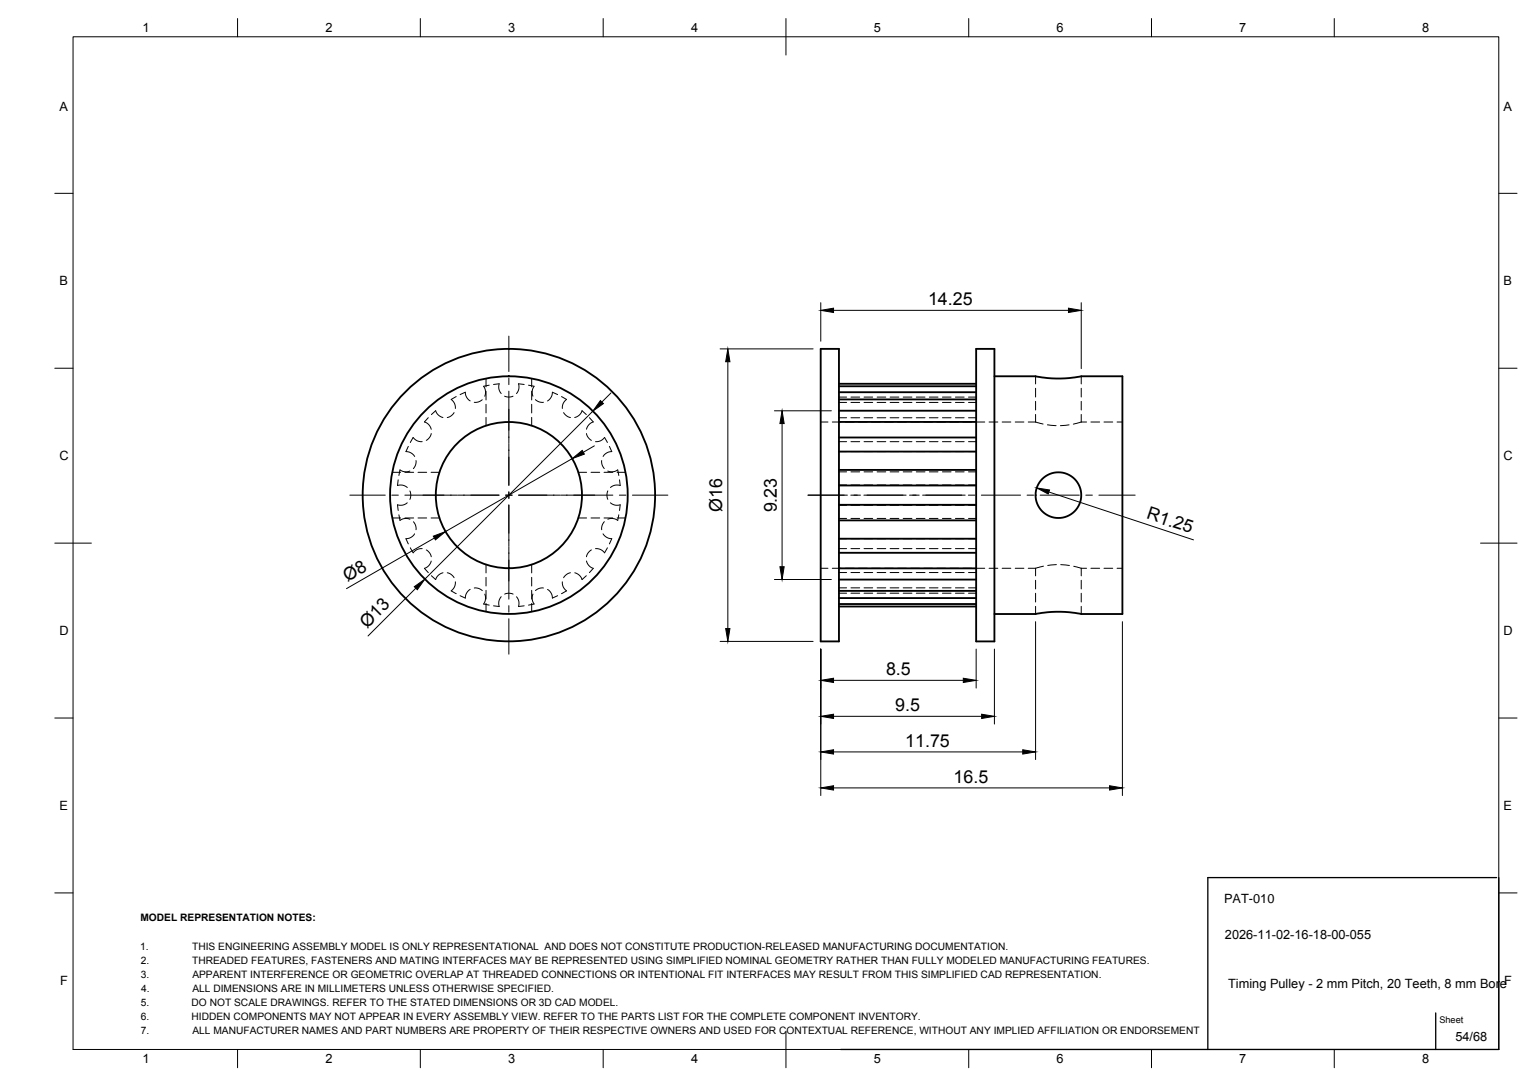
ISO-10303-21;
HEADER;
/* Generated by software containing ST-Developer
 * from STEP Tools, Inc. (www.steptools.com) 
 */

FILE_DESCRIPTION(
/* description */ ('Belt conveyor head drive unit'),
/* implementation_level */ '2;1');

FILE_NAME(
/* name */ 'Timing Pulley - 2 mm Pitch, 20 Teeth, 8 mm Bore.step',
/* time_stamp */ '2026-10-28T03:26:19-07:00',
/* author */ (''),
/* organization */ (''),
/* preprocessor_version */ 'ST-DEVELOPER v20.2',
/* originating_system */ 'Autodesk Translation Framework v15.17.0.0',
/* authorisation */ '');

FILE_SCHEMA (('AUTOMOTIVE_DESIGN { 1 0 10303 214 3 1 1 }'));
ENDSEC;

DATA;
#10=MECHANICAL_DESIGN_GEOMETRIC_PRESENTATION_REPRESENTATION('',(#915),#27069);
#585=B_SPLINE_CURVE_WITH_KNOTS('',3,(#24720,#24721,#24722,#24723,#24724,
#24725,#24726,#24727,#24728,#24729),.UNSPECIFIED.,.F.,.F.,(4,2,2,2,4),(0.566550474129931,
0.613761886174531,0.66097329821913,0.708186965196186,0.755400632173242),
 .UNSPECIFIED.);
#586=B_SPLINE_CURVE_WITH_KNOTS('',3,(#24731,#24732,#24733,#24734,#24735,
#24736,#24737,#24738,#24739,#24740,#24741,#24742,#24743,#24744,#24745,#24746,
#24747,#24748),.UNSPECIFIED.,.F.,.F.,(4,2,2,2,2,2,2,2,4),(0.18885015804331,
0.23606157008791,0.283272982132509,0.330486649109565,0.377700316086621,
0.424913983063677,0.472127650040732,0.519339062085332,0.566550474129931),
 .UNSPECIFIED.);
#587=B_SPLINE_CURVE_WITH_KNOTS('',3,(#24749,#24750,#24751,#24752,#24753,
#24754,#24755,#24756,#24757,#24758),.UNSPECIFIED.,.F.,.F.,(4,2,2,2,4),(0.755400632173242,
0.802614299150298,0.849827966127353,0.897039378171953,0.944250790216552),
 .UNSPECIFIED.);
#588=B_SPLINE_CURVE_WITH_KNOTS('',3,(#24762,#24763,#24764,#24765,#24766,
#24767,#24768,#24769,#24770,#24771),.UNSPECIFIED.,.F.,.F.,(4,2,2,2,4),(0.189723673274825,
0.237146208024627,0.28456874277443,0.33200804466204,0.37944734654965),
 .UNSPECIFIED.);
#589=B_SPLINE_CURVE_WITH_KNOTS('',3,(#24773,#24774,#24775,#24776,#24777,
#24778,#24779,#24780,#24781,#24782),.UNSPECIFIED.,.F.,.F.,(4,2,2,2,4),(0.,
0.0474393018876097,0.0948786037752193,0.142301138525022,0.189723673274825),
 .UNSPECIFIED.);
#590=B_SPLINE_CURVE_WITH_KNOTS('',3,(#24784,#24785,#24786,#24787,#24788,
#24789,#24790,#24791,#24792,#24793),.UNSPECIFIED.,.F.,.F.,(4,2,2,2,4),(0.569171019824474,
0.616593554574277,0.66401608932408,0.711455391211689,0.758894693099299),
 .UNSPECIFIED.);
#591=B_SPLINE_CURVE_WITH_KNOTS('',3,(#24794,#24795,#24796,#24797,#24798,
#24799,#24800,#24801,#24802,#24803),.UNSPECIFIED.,.F.,.F.,(4,2,2,2,4),(0.37944734654965,
0.426886648437259,0.474325950324869,0.521748485074671,0.569171019824474),
 .UNSPECIFIED.);
#592=B_SPLINE_CURVE_WITH_KNOTS('',3,(#24807,#24808,#24809,#24810,#24811,
#24812,#24813,#24814,#24815,#24816,#24817,#24818,#24819,#24820,#24821,#24822,
#24823,#24824),.UNSPECIFIED.,.F.,.F.,(4,2,2,2,2,2,2,2,4),(0.,0.0474393018876097,
0.0948786037752194,0.142301138525022,0.189723673274825,0.237146208024628,
0.28456874277443,0.33200804466204,0.37944734654965),.UNSPECIFIED.);
#593=B_SPLINE_CURVE_WITH_KNOTS('',3,(#24825,#24826,#24827,#24828,#24829,
#24830,#24831,#24832,#24833,#24834,#24835,#24836,#24837,#24838,#24839,#24840,
#24841,#24842),.UNSPECIFIED.,.F.,.F.,(4,2,2,2,2,2,2,2,4),(0.37944734654965,
0.426886648437259,0.474325950324869,0.521748485074672,0.569171019824474,
0.616593554574277,0.66401608932408,0.711455391211689,0.758894693099299),
 .UNSPECIFIED.);
#594=B_SPLINE_CURVE_WITH_KNOTS('',3,(#24846,#24847,#24848,#24849,#24850,
#24851,#24852,#24853,#24854,#24855),.UNSPECIFIED.,.F.,.F.,(4,2,2,2,4),(0.566550474129931,
0.613761886174531,0.66097329821913,0.708186965196186,0.755400632173242),
 .UNSPECIFIED.);
#595=B_SPLINE_CURVE_WITH_KNOTS('',3,(#24857,#24858,#24859,#24860,#24861,
#24862,#24863,#24864,#24865,#24866,#24867,#24868,#24869,#24870,#24871,#24872,
#24873,#24874),.UNSPECIFIED.,.F.,.F.,(4,2,2,2,2,2,2,2,4),(0.188850158043311,
0.23606157008791,0.283272982132509,0.330486649109565,0.377700316086621,
0.424913983063677,0.472127650040733,0.519339062085332,0.566550474129931),
 .UNSPECIFIED.);
#596=B_SPLINE_CURVE_WITH_KNOTS('',3,(#24875,#24876,#24877,#24878,#24879,
#24880,#24881,#24882,#24883,#24884),.UNSPECIFIED.,.F.,.F.,(4,2,2,2,4),(0.755400632173242,
0.802614299150298,0.849827966127354,0.897039378171953,0.944250790216552),
 .UNSPECIFIED.);
#597=B_SPLINE_CURVE_WITH_KNOTS('',3,(#24894,#24895,#24896,#24897,#24898,
#24899,#24900,#24901,#24902,#24903,#24904,#24905,#24906,#24907,#24908,#24909,
#24910,#24911),.UNSPECIFIED.,.F.,.F.,(4,2,2,2,2,2,2,2,4),(0.18885015804331,
0.23606157008791,0.283272982132509,0.330486649109565,0.377700316086621,
0.424913983063677,0.472127650040732,0.519339062085332,0.566550474129931),
 .UNSPECIFIED.);
#598=B_SPLINE_CURVE_WITH_KNOTS('',3,(#24913,#24914,#24915,#24916,#24917,
#24918,#24919,#24920,#24921,#24922),.UNSPECIFIED.,.F.,.F.,(4,2,2,2,4),(0.566550474129931,
0.613761886174531,0.66097329821913,0.708186965196186,0.755400632173242),
 .UNSPECIFIED.);
#599=B_SPLINE_CURVE_WITH_KNOTS('',3,(#24923,#24924,#24925,#24926,#24927,
#24928,#24929,#24930,#24931,#24932),.UNSPECIFIED.,.F.,.F.,(4,2,2,2,4),(0.755400632173242,
0.802614299150298,0.849827966127353,0.897039378171953,0.944250790216552),
 .UNSPECIFIED.);
#600=B_SPLINE_CURVE_WITH_KNOTS('',3,(#24935,#24936,#24937,#24938,#24939,
#24940,#24941,#24942,#24943,#24944,#24945,#24946,#24947,#24948,#24949,#24950,
#24951,#24952),.UNSPECIFIED.,.F.,.F.,(4,2,2,2,2,2,2,2,4),(0.188850158043311,
0.23606157008791,0.283272982132509,0.330486649109565,0.377700316086621,
0.424913983063677,0.472127650040733,0.519339062085332,0.566550474129932),
 .UNSPECIFIED.);
#601=B_SPLINE_CURVE_WITH_KNOTS('',3,(#24954,#24955,#24956,#24957,#24958,
#24959,#24960,#24961,#24962,#24963),.UNSPECIFIED.,.F.,.F.,(4,2,2,2,4),(0.566550474129932,
0.613761886174531,0.66097329821913,0.708186965196186,0.755400632173242),
 .UNSPECIFIED.);
#602=B_SPLINE_CURVE_WITH_KNOTS('',3,(#24964,#24965,#24966,#24967,#24968,
#24969,#24970,#24971,#24972,#24973),.UNSPECIFIED.,.F.,.F.,(4,2,2,2,4),(0.755400632173242,
0.802614299150298,0.849827966127354,0.897039378171953,0.944250790216552),
 .UNSPECIFIED.);
#603=B_SPLINE_CURVE_WITH_KNOTS('',3,(#24978,#24979,#24980,#24981,#24982,
#24983,#24984,#24985,#24986,#24987,#24988,#24989,#24990,#24991,#24992,#24993,
#24994,#24995),.UNSPECIFIED.,.F.,.F.,(4,2,2,2,2,2,2,2,4),(0.,0.0474393018876097,
0.0948786037752193,0.142301138525022,0.189723673274825,0.237146208024627,
0.28456874277443,0.33200804466204,0.37944734654965),.UNSPECIFIED.);
#604=B_SPLINE_CURVE_WITH_KNOTS('',3,(#24996,#24997,#24998,#24999,#25000,
#25001,#25002,#25003,#25004,#25005,#25006,#25007,#25008,#25009,#25010,#25011,
#25012,#25013),.UNSPECIFIED.,.F.,.F.,(4,2,2,2,2,2,2,2,4),(0.37944734654965,
0.426886648437259,0.474325950324869,0.521748485074672,0.569171019824474,
0.616593554574277,0.66401608932408,0.711455391211689,0.758894693099299),
 .UNSPECIFIED.);
#605=B_SPLINE_CURVE_WITH_KNOTS('',3,(#25017,#25018,#25019,#25020,#25021,
#25022,#25023,#25024,#25025,#25026,#25027,#25028,#25029,#25030,#25031,#25032,
#25033,#25034),.UNSPECIFIED.,.F.,.F.,(4,2,2,2,2,2,2,2,4),(0.,0.0474393018876097,
0.0948786037752194,0.142301138525022,0.189723673274825,0.237146208024627,
0.28456874277443,0.33200804466204,0.37944734654965),.UNSPECIFIED.);
#606=B_SPLINE_CURVE_WITH_KNOTS('',3,(#25035,#25036,#25037,#25038,#25039,
#25040,#25041,#25042,#25043,#25044,#25045,#25046,#25047,#25048,#25049,#25050,
#25051,#25052),.UNSPECIFIED.,.F.,.F.,(4,2,2,2,2,2,2,2,4),(0.37944734654965,
0.426886648437259,0.474325950324869,0.521748485074672,0.569171019824474,
0.616593554574277,0.66401608932408,0.711455391211689,0.758894693099299),
 .UNSPECIFIED.);
#761=SHAPE_REPRESENTATION_RELATIONSHIP('SRR','None',#27409,#830);
#830=ADVANCED_BREP_SHAPE_REPRESENTATION('',(#996),#27051);
#915=STYLED_ITEM('',(#27811),#996);
#996=MANIFOLD_SOLID_BREP('Body1',#13784);
#1222=FACE_BOUND('',#3204,.T.);
#1223=FACE_BOUND('',#3205,.T.);
#1224=FACE_BOUND('',#3206,.T.);
#1225=FACE_BOUND('',#3210,.T.);
#1226=FACE_BOUND('',#3211,.T.);
#1227=FACE_BOUND('',#3212,.T.);
#1228=FACE_BOUND('',#3214,.T.);
#1229=FACE_BOUND('',#3216,.T.);
#1230=FACE_BOUND('',#3219,.T.);
#1231=FACE_BOUND('',#3221,.T.);
#1232=FACE_BOUND('',#3224,.T.);
#1566=PLANE('',#15740);
#1567=PLANE('',#15741);
#1568=PLANE('',#15785);
#1569=PLANE('',#15786);
#1570=PLANE('',#15830);
#2191=FACE_OUTER_BOUND('',#3201,.T.);
#2192=FACE_OUTER_BOUND('',#3202,.T.);
#2193=FACE_OUTER_BOUND('',#3203,.T.);
#2194=FACE_OUTER_BOUND('',#3207,.T.);
#2195=FACE_OUTER_BOUND('',#3208,.T.);
#2196=FACE_OUTER_BOUND('',#3209,.T.);
#2197=FACE_OUTER_BOUND('',#3213,.T.);
#2198=FACE_OUTER_BOUND('',#3215,.T.);
#2199=FACE_OUTER_BOUND('',#3217,.T.);
#2200=FACE_OUTER_BOUND('',#3218,.T.);
#2201=FACE_OUTER_BOUND('',#3220,.T.);
#2202=FACE_OUTER_BOUND('',#3222,.T.);
#2203=FACE_OUTER_BOUND('',#3223,.T.);
#2204=FACE_OUTER_BOUND('',#3225,.T.);
#2205=FACE_OUTER_BOUND('',#3226,.T.);
#2206=FACE_OUTER_BOUND('',#3227,.T.);
#2207=FACE_OUTER_BOUND('',#3228,.T.);
#2208=FACE_OUTER_BOUND('',#3229,.T.);
#2209=FACE_OUTER_BOUND('',#3230,.T.);
#2210=FACE_OUTER_BOUND('',#3231,.T.);
#2211=FACE_OUTER_BOUND('',#3232,.T.);
#2212=FACE_OUTER_BOUND('',#3233,.T.);
#2213=FACE_OUTER_BOUND('',#3234,.T.);
#2214=FACE_OUTER_BOUND('',#3235,.T.);
#2215=FACE_OUTER_BOUND('',#3236,.T.);
#2216=FACE_OUTER_BOUND('',#3237,.T.);
#2217=FACE_OUTER_BOUND('',#3238,.T.);
#2218=FACE_OUTER_BOUND('',#3239,.T.);
#2219=FACE_OUTER_BOUND('',#3240,.T.);
#2220=FACE_OUTER_BOUND('',#3241,.T.);
#2221=FACE_OUTER_BOUND('',#3242,.T.);
#2222=FACE_OUTER_BOUND('',#3243,.T.);
#2223=FACE_OUTER_BOUND('',#3244,.T.);
#2224=FACE_OUTER_BOUND('',#3245,.T.);
#2225=FACE_OUTER_BOUND('',#3246,.T.);
#2226=FACE_OUTER_BOUND('',#3247,.T.);
#2227=FACE_OUTER_BOUND('',#3248,.T.);
#2228=FACE_OUTER_BOUND('',#3249,.T.);
#2229=FACE_OUTER_BOUND('',#3250,.T.);
#2230=FACE_OUTER_BOUND('',#3251,.T.);
#2231=FACE_OUTER_BOUND('',#3252,.T.);
#2232=FACE_OUTER_BOUND('',#3253,.T.);
#2233=FACE_OUTER_BOUND('',#3254,.T.);
#2234=FACE_OUTER_BOUND('',#3255,.T.);
#2235=FACE_OUTER_BOUND('',#3256,.T.);
#2236=FACE_OUTER_BOUND('',#3257,.T.);
#2237=FACE_OUTER_BOUND('',#3258,.T.);
#2238=FACE_OUTER_BOUND('',#3259,.T.);
#2239=FACE_OUTER_BOUND('',#3260,.T.);
#2240=FACE_OUTER_BOUND('',#3261,.T.);
#2241=FACE_OUTER_BOUND('',#3262,.T.);
#2242=FACE_OUTER_BOUND('',#3263,.T.);
#2243=FACE_OUTER_BOUND('',#3264,.T.);
#3201=EDGE_LOOP('',(#11302,#11303,#11304,#11305,#11306,#11307,#11308,#11309,
#11310));
#3202=EDGE_LOOP('',(#11311,#11312,#11313,#11314,#11315,#11316,#11317));
#3203=EDGE_LOOP('',(#11318,#11319,#11320,#11321,#11322,#11323,#11324,#11325,
#11326));
#3204=EDGE_LOOP('',(#11327,#11328,#11329));
#3205=EDGE_LOOP('',(#11330,#11331,#11332));
#3206=EDGE_LOOP('',(#11333,#11334,#11335));
#3207=EDGE_LOOP('',(#11336,#11337,#11338,#11339,#11340,#11341,#11342));
#3208=EDGE_LOOP('',(#11343,#11344,#11345,#11346,#11347,#11348,#11349));
#3209=EDGE_LOOP('',(#11350,#11351,#11352,#11353,#11354,#11355,#11356,#11357,
#11358,#11359));
#3210=EDGE_LOOP('',(#11360,#11361));
#3211=EDGE_LOOP('',(#11362,#11363));
#3212=EDGE_LOOP('',(#11364,#11365));
#3213=EDGE_LOOP('',(#11366));
#3214=EDGE_LOOP('',(#11367));
#3215=EDGE_LOOP('',(#11368));
#3216=EDGE_LOOP('',(#11369,#11370,#11371,#11372,#11373,#11374,#11375,#11376,
#11377,#11378,#11379,#11380,#11381,#11382,#11383,#11384,#11385,#11386,#11387,
#11388,#11389,#11390,#11391,#11392,#11393,#11394,#11395,#11396,#11397,#11398,
#11399,#11400,#11401,#11402,#11403,#11404,#11405,#11406,#11407,#11408));
#3217=EDGE_LOOP('',(#11409,#11410,#11411,#11412));
#3218=EDGE_LOOP('',(#11413));
#3219=EDGE_LOOP('',(#11414));
#3220=EDGE_LOOP('',(#11415));
#3221=EDGE_LOOP('',(#11416,#11417,#11418,#11419,#11420,#11421,#11422,#11423,
#11424,#11425,#11426,#11427,#11428,#11429,#11430,#11431,#11432,#11433,#11434,
#11435,#11436,#11437,#11438,#11439,#11440,#11441,#11442,#11443,#11444,#11445,
#11446,#11447,#11448,#11449,#11450,#11451,#11452,#11453,#11454,#11455));
#3222=EDGE_LOOP('',(#11456,#11457,#11458,#11459));
#3223=EDGE_LOOP('',(#11460));
#3224=EDGE_LOOP('',(#11461));
#3225=EDGE_LOOP('',(#11462,#11463,#11464,#11465));
#3226=EDGE_LOOP('',(#11466,#11467,#11468,#11469));
#3227=EDGE_LOOP('',(#11470,#11471,#11472,#11473));
#3228=EDGE_LOOP('',(#11474,#11475,#11476,#11477));
#3229=EDGE_LOOP('',(#11478,#11479,#11480,#11481));
#3230=EDGE_LOOP('',(#11482,#11483,#11484,#11485));
#3231=EDGE_LOOP('',(#11486,#11487,#11488,#11489));
#3232=EDGE_LOOP('',(#11490,#11491,#11492,#11493));
#3233=EDGE_LOOP('',(#11494,#11495,#11496,#11497));
#3234=EDGE_LOOP('',(#11498,#11499,#11500,#11501));
#3235=EDGE_LOOP('',(#11502,#11503,#11504,#11505));
#3236=EDGE_LOOP('',(#11506,#11507,#11508,#11509));
#3237=EDGE_LOOP('',(#11510,#11511,#11512,#11513));
#3238=EDGE_LOOP('',(#11514,#11515,#11516,#11517));
#3239=EDGE_LOOP('',(#11518,#11519,#11520,#11521));
#3240=EDGE_LOOP('',(#11522,#11523,#11524,#11525));
#3241=EDGE_LOOP('',(#11526,#11527,#11528,#11529));
#3242=EDGE_LOOP('',(#11530,#11531,#11532,#11533));
#3243=EDGE_LOOP('',(#11534,#11535,#11536,#11537));
#3244=EDGE_LOOP('',(#11538,#11539,#11540,#11541));
#3245=EDGE_LOOP('',(#11542,#11543,#11544,#11545));
#3246=EDGE_LOOP('',(#11546,#11547,#11548,#11549));
#3247=EDGE_LOOP('',(#11550,#11551,#11552,#11553));
#3248=EDGE_LOOP('',(#11554,#11555,#11556,#11557));
#3249=EDGE_LOOP('',(#11558,#11559,#11560,#11561));
#3250=EDGE_LOOP('',(#11562,#11563,#11564,#11565));
#3251=EDGE_LOOP('',(#11566,#11567,#11568,#11569));
#3252=EDGE_LOOP('',(#11570,#11571,#11572,#11573));
#3253=EDGE_LOOP('',(#11574,#11575,#11576,#11577));
#3254=EDGE_LOOP('',(#11578,#11579,#11580,#11581));
#3255=EDGE_LOOP('',(#11582,#11583,#11584,#11585));
#3256=EDGE_LOOP('',(#11586,#11587,#11588,#11589));
#3257=EDGE_LOOP('',(#11590,#11591,#11592,#11593));
#3258=EDGE_LOOP('',(#11594,#11595,#11596,#11597));
#3259=EDGE_LOOP('',(#11598,#11599,#11600,#11601));
#3260=EDGE_LOOP('',(#11602,#11603,#11604,#11605));
#3261=EDGE_LOOP('',(#11606,#11607,#11608,#11609));
#3262=EDGE_LOOP('',(#11610,#11611,#11612,#11613));
#3263=EDGE_LOOP('',(#11614,#11615,#11616,#11617));
#3264=EDGE_LOOP('',(#11618,#11619,#11620,#11621));
#4067=LINE('',#24760,#4859);
#4068=LINE('',#24844,#4860);
#4069=LINE('',#24888,#4861);
#4070=LINE('',#24890,#4862);
#4071=LINE('',#24976,#4863);
#4072=LINE('',#25053,#4864);
#4073=LINE('',#25057,#4865);
#4074=LINE('',#25059,#4866);
#4075=LINE('',#25148,#4867);
#4076=LINE('',#25236,#4868);
#4077=LINE('',#25239,#4869);
#4078=LINE('',#25240,#4870);
#4079=LINE('',#25242,#4871);
#4080=LINE('',#25244,#4872);
#4081=LINE('',#25246,#4873);
#4082=LINE('',#25248,#4874);
#4083=LINE('',#25250,#4875);
#4084=LINE('',#25252,#4876);
#4085=LINE('',#25254,#4877);
#4086=LINE('',#25256,#4878);
#4087=LINE('',#25258,#4879);
#4088=LINE('',#25260,#4880);
#4089=LINE('',#25262,#4881);
#4090=LINE('',#25264,#4882);
#4091=LINE('',#25266,#4883);
#4092=LINE('',#25268,#4884);
#4093=LINE('',#25270,#4885);
#4094=LINE('',#25272,#4886);
#4095=LINE('',#25274,#4887);
#4096=LINE('',#25276,#4888);
#4097=LINE('',#25278,#4889);
#4098=LINE('',#25280,#4890);
#4099=LINE('',#25282,#4891);
#4100=LINE('',#25284,#4892);
#4101=LINE('',#25286,#4893);
#4102=LINE('',#25288,#4894);
#4103=LINE('',#25290,#4895);
#4104=LINE('',#25292,#4896);
#4105=LINE('',#25294,#4897);
#4106=LINE('',#25296,#4898);
#4107=LINE('',#25298,#4899);
#4108=LINE('',#25300,#4900);
#4109=LINE('',#25302,#4901);
#4110=LINE('',#25304,#4902);
#4111=LINE('',#25306,#4903);
#4112=LINE('',#25308,#4904);
#4113=LINE('',#25310,#4905);
#4114=LINE('',#25312,#4906);
#4115=LINE('',#25314,#4907);
#4116=LINE('',#25316,#4908);
#4859=VECTOR('',#19341,0.125);
#4860=VECTOR('',#19344,0.125);
#4861=VECTOR('',#19349,0.65);
#4862=VECTOR('',#19350,0.65);
#4863=VECTOR('',#19355,0.125);
#4864=VECTOR('',#19358,0.125);
#4865=VECTOR('',#19363,0.4);
#4866=VECTOR('',#19364,0.4);
#4867=VECTOR('',#19457,0.8);
#4868=VECTOR('',#19548,0.8);
#4869=VECTOR('',#19553,1.);
#4870=VECTOR('',#19554,1.);
#4871=VECTOR('',#19557,1.);
#4872=VECTOR('',#19560,1.);
#4873=VECTOR('',#19563,1.);
#4874=VECTOR('',#19566,1.);
#4875=VECTOR('',#19569,1.);
#4876=VECTOR('',#19572,1.);
#4877=VECTOR('',#19575,1.);
#4878=VECTOR('',#19578,1.);
#4879=VECTOR('',#19581,1.);
#4880=VECTOR('',#19584,1.);
#4881=VECTOR('',#19587,1.);
#4882=VECTOR('',#19590,1.);
#4883=VECTOR('',#19593,1.);
#4884=VECTOR('',#19596,1.);
#4885=VECTOR('',#19599,1.);
#4886=VECTOR('',#19602,1.);
#4887=VECTOR('',#19605,1.);
#4888=VECTOR('',#19608,1.);
#4889=VECTOR('',#19611,1.);
#4890=VECTOR('',#19614,1.);
#4891=VECTOR('',#19617,1.);
#4892=VECTOR('',#19620,1.);
#4893=VECTOR('',#19623,1.);
#4894=VECTOR('',#19626,1.);
#4895=VECTOR('',#19629,1.);
#4896=VECTOR('',#19632,1.);
#4897=VECTOR('',#19635,1.);
#4898=VECTOR('',#19638,1.);
#4899=VECTOR('',#19641,1.);
#4900=VECTOR('',#19644,1.);
#4901=VECTOR('',#19647,1.);
#4902=VECTOR('',#19650,1.);
#4903=VECTOR('',#19653,1.);
#4904=VECTOR('',#19656,1.);
#4905=VECTOR('',#19659,1.);
#4906=VECTOR('',#19662,1.);
#4907=VECTOR('',#19665,1.);
#4908=VECTOR('',#19668,1.);
#5621=CIRCLE('',#15733,0.65);
#5622=CIRCLE('',#15734,0.65);
#5623=CIRCLE('',#15738,0.4);
#5624=CIRCLE('',#15739,0.4);
#5625=CIRCLE('',#15742,0.8);
#5626=CIRCLE('',#15743,0.0555);
#5627=CIRCLE('',#15744,0.611219772367581);
#5628=CIRCLE('',#15745,0.0555);
#5629=CIRCLE('',#15746,0.611219772367581);
#5630=CIRCLE('',#15747,0.0555);
#5631=CIRCLE('',#15748,0.611219772367581);
#5632=CIRCLE('',#15749,0.0555);
#5633=CIRCLE('',#15750,0.611219772367581);
#5634=CIRCLE('',#15751,0.0555);
#5635=CIRCLE('',#15752,0.611219772367581);
#5636=CIRCLE('',#15753,0.0555);
#5637=CIRCLE('',#15754,0.611219772367581);
#5638=CIRCLE('',#15755,0.0555);
#5639=CIRCLE('',#15756,0.611219772367581);
#5640=CIRCLE('',#15757,0.0555);
#5641=CIRCLE('',#15758,0.611219772367581);
#5642=CIRCLE('',#15759,0.0555);
#5643=CIRCLE('',#15760,0.611219772367581);
#5644=CIRCLE('',#15761,0.0555);
#5645=CIRCLE('',#15762,0.611219772367581);
#5646=CIRCLE('',#15763,0.0555);
#5647=CIRCLE('',#15764,0.611219772367581);
#5648=CIRCLE('',#15765,0.0555);
#5649=CIRCLE('',#15766,0.611219772367581);
#5650=CIRCLE('',#15767,0.0555);
#5651=CIRCLE('',#15768,0.611219772367581);
#5652=CIRCLE('',#15769,0.0555);
#5653=CIRCLE('',#15770,0.611219772367581);
#5654=CIRCLE('',#15771,0.0555);
#5655=CIRCLE('',#15772,0.611219772367581);
#5656=CIRCLE('',#15773,0.0555);
#5657=CIRCLE('',#15774,0.611219772367581);
#5658=CIRCLE('',#15775,0.0555);
#5659=CIRCLE('',#15776,0.611219772367581);
#5660=CIRCLE('',#15777,0.0555);
#5661=CIRCLE('',#15778,0.611219772367581);
#5662=CIRCLE('',#15779,0.0555);
#5663=CIRCLE('',#15780,0.611219772367581);
#5664=CIRCLE('',#15781,0.0555);
#5665=CIRCLE('',#15782,0.611219772367581);
#5666=CIRCLE('',#15784,0.8);
#5667=CIRCLE('',#15787,0.8);
#5668=CIRCLE('',#15788,0.0555);
#5669=CIRCLE('',#15789,0.611219772367581);
#5670=CIRCLE('',#15790,0.0555);
#5671=CIRCLE('',#15791,0.611219772367581);
#5672=CIRCLE('',#15792,0.0555);
#5673=CIRCLE('',#15793,0.611219772367581);
#5674=CIRCLE('',#15794,0.0555);
#5675=CIRCLE('',#15795,0.611219772367581);
#5676=CIRCLE('',#15796,0.0555);
#5677=CIRCLE('',#15797,0.611219772367581);
#5678=CIRCLE('',#15798,0.0555);
#5679=CIRCLE('',#15799,0.611219772367581);
#5680=CIRCLE('',#15800,0.0555);
#5681=CIRCLE('',#15801,0.611219772367581);
#5682=CIRCLE('',#15802,0.0555);
#5683=CIRCLE('',#15803,0.611219772367581);
#5684=CIRCLE('',#15804,0.0555);
#5685=CIRCLE('',#15805,0.611219772367581);
#5686=CIRCLE('',#15806,0.0555);
#5687=CIRCLE('',#15807,0.611219772367581);
#5688=CIRCLE('',#15808,0.0555);
#5689=CIRCLE('',#15809,0.611219772367581);
#5690=CIRCLE('',#15810,0.0555);
#5691=CIRCLE('',#15811,0.611219772367581);
#5692=CIRCLE('',#15812,0.0555);
#5693=CIRCLE('',#15813,0.611219772367581);
#5694=CIRCLE('',#15814,0.0555);
#5695=CIRCLE('',#15815,0.611219772367581);
#5696=CIRCLE('',#15816,0.0555);
#5697=CIRCLE('',#15817,0.611219772367581);
#5698=CIRCLE('',#15818,0.0555);
#5699=CIRCLE('',#15819,0.611219772367581);
#5700=CIRCLE('',#15820,0.0555);
#5701=CIRCLE('',#15821,0.611219772367581);
#5702=CIRCLE('',#15822,0.0555);
#5703=CIRCLE('',#15823,0.611219772367581);
#5704=CIRCLE('',#15824,0.0555);
#5705=CIRCLE('',#15825,0.611219772367581);
#5706=CIRCLE('',#15826,0.0555);
#5707=CIRCLE('',#15827,0.611219772367581);
#5708=CIRCLE('',#15829,0.8);
#6755=VERTEX_POINT('',#24718);
#6756=VERTEX_POINT('',#24719);
#6757=VERTEX_POINT('',#24730);
#6758=VERTEX_POINT('',#24759);
#6759=VERTEX_POINT('',#24761);
#6760=VERTEX_POINT('',#24772);
#6761=VERTEX_POINT('',#24783);
#6762=VERTEX_POINT('',#24805);
#6763=VERTEX_POINT('',#24806);
#6764=VERTEX_POINT('',#24843);
#6765=VERTEX_POINT('',#24845);
#6766=VERTEX_POINT('',#24856);
#6767=VERTEX_POINT('',#24886);
#6768=VERTEX_POINT('',#24889);
#6769=VERTEX_POINT('',#24892);
#6770=VERTEX_POINT('',#24893);
#6771=VERTEX_POINT('',#24912);
#6772=VERTEX_POINT('',#24933);
#6773=VERTEX_POINT('',#24934);
#6774=VERTEX_POINT('',#24953);
#6775=VERTEX_POINT('',#24975);
#6776=VERTEX_POINT('',#24977);
#6777=VERTEX_POINT('',#25015);
#6778=VERTEX_POINT('',#25016);
#6779=VERTEX_POINT('',#25055);
#6780=VERTEX_POINT('',#25058);
#6781=VERTEX_POINT('',#25063);
#6782=VERTEX_POINT('',#25065);
#6783=VERTEX_POINT('',#25066);
#6784=VERTEX_POINT('',#25068);
#6785=VERTEX_POINT('',#25070);
#6786=VERTEX_POINT('',#25072);
#6787=VERTEX_POINT('',#25074);
#6788=VERTEX_POINT('',#25076);
#6789=VERTEX_POINT('',#25078);
#6790=VERTEX_POINT('',#25080);
#6791=VERTEX_POINT('',#25082);
#6792=VERTEX_POINT('',#25084);
#6793=VERTEX_POINT('',#25086);
#6794=VERTEX_POINT('',#25088);
#6795=VERTEX_POINT('',#25090);
#6796=VERTEX_POINT('',#25092);
#6797=VERTEX_POINT('',#25094);
#6798=VERTEX_POINT('',#25096);
#6799=VERTEX_POINT('',#25098);
#6800=VERTEX_POINT('',#25100);
#6801=VERTEX_POINT('',#25102);
#6802=VERTEX_POINT('',#25104);
#6803=VERTEX_POINT('',#25106);
#6804=VERTEX_POINT('',#25108);
#6805=VERTEX_POINT('',#25110);
#6806=VERTEX_POINT('',#25112);
#6807=VERTEX_POINT('',#25114);
#6808=VERTEX_POINT('',#25116);
#6809=VERTEX_POINT('',#25118);
#6810=VERTEX_POINT('',#25120);
#6811=VERTEX_POINT('',#25122);
#6812=VERTEX_POINT('',#25124);
#6813=VERTEX_POINT('',#25126);
#6814=VERTEX_POINT('',#25128);
#6815=VERTEX_POINT('',#25130);
#6816=VERTEX_POINT('',#25132);
#6817=VERTEX_POINT('',#25134);
#6818=VERTEX_POINT('',#25136);
#6819=VERTEX_POINT('',#25138);
#6820=VERTEX_POINT('',#25140);
#6821=VERTEX_POINT('',#25142);
#6822=VERTEX_POINT('',#25146);
#6823=VERTEX_POINT('',#25151);
#6824=VERTEX_POINT('',#25153);
#6825=VERTEX_POINT('',#25154);
#6826=VERTEX_POINT('',#25156);
#6827=VERTEX_POINT('',#25158);
#6828=VERTEX_POINT('',#25160);
#6829=VERTEX_POINT('',#25162);
#6830=VERTEX_POINT('',#25164);
#6831=VERTEX_POINT('',#25166);
#6832=VERTEX_POINT('',#25168);
#6833=VERTEX_POINT('',#25170);
#6834=VERTEX_POINT('',#25172);
#6835=VERTEX_POINT('',#25174);
#6836=VERTEX_POINT('',#25176);
#6837=VERTEX_POINT('',#25178);
#6838=VERTEX_POINT('',#25180);
#6839=VERTEX_POINT('',#25182);
#6840=VERTEX_POINT('',#25184);
#6841=VERTEX_POINT('',#25186);
#6842=VERTEX_POINT('',#25188);
#6843=VERTEX_POINT('',#25190);
#6844=VERTEX_POINT('',#25192);
#6845=VERTEX_POINT('',#25194);
#6846=VERTEX_POINT('',#25196);
#6847=VERTEX_POINT('',#25198);
#6848=VERTEX_POINT('',#25200);
#6849=VERTEX_POINT('',#25202);
#6850=VERTEX_POINT('',#25204);
#6851=VERTEX_POINT('',#25206);
#6852=VERTEX_POINT('',#25208);
#6853=VERTEX_POINT('',#25210);
#6854=VERTEX_POINT('',#25212);
#6855=VERTEX_POINT('',#25214);
#6856=VERTEX_POINT('',#25216);
#6857=VERTEX_POINT('',#25218);
#6858=VERTEX_POINT('',#25220);
#6859=VERTEX_POINT('',#25222);
#6860=VERTEX_POINT('',#25224);
#6861=VERTEX_POINT('',#25226);
#6862=VERTEX_POINT('',#25228);
#6863=VERTEX_POINT('',#25230);
#6864=VERTEX_POINT('',#25234);
#8343=EDGE_CURVE('',#6755,#6756,#585,.T.);
#8344=EDGE_CURVE('',#6757,#6755,#586,.T.);
#8345=EDGE_CURVE('',#6756,#6757,#587,.T.);
#8346=EDGE_CURVE('',#6756,#6758,#4067,.T.);
#8347=EDGE_CURVE('',#6759,#6758,#588,.T.);
#8348=EDGE_CURVE('',#6760,#6759,#589,.T.);
#8349=EDGE_CURVE('',#6761,#6760,#590,.T.);
#8350=EDGE_CURVE('',#6758,#6761,#591,.T.);
#8351=EDGE_CURVE('',#6762,#6763,#592,.T.);
#8352=EDGE_CURVE('',#6763,#6762,#593,.T.);
#8353=EDGE_CURVE('',#6763,#6764,#4068,.T.);
#8354=EDGE_CURVE('',#6765,#6764,#594,.T.);
#8355=EDGE_CURVE('',#6766,#6765,#595,.T.);
#8356=EDGE_CURVE('',#6764,#6766,#596,.T.);
#8357=EDGE_CURVE('',#6767,#6767,#5621,.T.);
#8358=EDGE_CURVE('',#6767,#6757,#4069,.T.);
#8359=EDGE_CURVE('',#6755,#6768,#4070,.T.);
#8360=EDGE_CURVE('',#6768,#6768,#5622,.T.);
#8361=EDGE_CURVE('',#6769,#6770,#597,.T.);
#8362=EDGE_CURVE('',#6770,#6771,#598,.T.);
#8363=EDGE_CURVE('',#6771,#6769,#599,.T.);
#8364=EDGE_CURVE('',#6772,#6773,#600,.T.);
#8365=EDGE_CURVE('',#6773,#6774,#601,.T.);
#8366=EDGE_CURVE('',#6774,#6772,#602,.T.);
#8367=EDGE_CURVE('',#6771,#6775,#4071,.T.);
#8368=EDGE_CURVE('',#6776,#6775,#603,.T.);
#8369=EDGE_CURVE('',#6775,#6776,#604,.T.);
#8370=EDGE_CURVE('',#6777,#6778,#605,.T.);
#8371=EDGE_CURVE('',#6778,#6777,#606,.T.);
#8372=EDGE_CURVE('',#6778,#6774,#4072,.T.);
#8373=EDGE_CURVE('',#6779,#6779,#5623,.T.);
#8374=EDGE_CURVE('',#6779,#6759,#4073,.T.);
#8375=EDGE_CURVE('',#6761,#6780,#4074,.T.);
#8376=EDGE_CURVE('',#6780,#6780,#5624,.T.);
#8377=EDGE_CURVE('',#6781,#6781,#5625,.T.);
#8378=EDGE_CURVE('',#6782,#6783,#5626,.T.);
#8379=EDGE_CURVE('',#6784,#6783,#5627,.T.);
#8380=EDGE_CURVE('',#6784,#6785,#5628,.T.);
#8381=EDGE_CURVE('',#6786,#6785,#5629,.T.);
#8382=EDGE_CURVE('',#6786,#6787,#5630,.T.);
#8383=EDGE_CURVE('',#6788,#6787,#5631,.T.);
#8384=EDGE_CURVE('',#6788,#6789,#5632,.T.);
#8385=EDGE_CURVE('',#6790,#6789,#5633,.T.);
#8386=EDGE_CURVE('',#6790,#6791,#5634,.T.);
#8387=EDGE_CURVE('',#6792,#6791,#5635,.T.);
#8388=EDGE_CURVE('',#6792,#6793,#5636,.T.);
#8389=EDGE_CURVE('',#6794,#6793,#5637,.T.);
#8390=EDGE_CURVE('',#6794,#6795,#5638,.T.);
#8391=EDGE_CURVE('',#6796,#6795,#5639,.T.);
#8392=EDGE_CURVE('',#6796,#6797,#5640,.T.);
#8393=EDGE_CURVE('',#6798,#6797,#5641,.T.);
#8394=EDGE_CURVE('',#6798,#6799,#5642,.T.);
#8395=EDGE_CURVE('',#6800,#6799,#5643,.T.);
#8396=EDGE_CURVE('',#6800,#6801,#5644,.T.);
#8397=EDGE_CURVE('',#6802,#6801,#5645,.T.);
#8398=EDGE_CURVE('',#6802,#6803,#5646,.T.);
#8399=EDGE_CURVE('',#6804,#6803,#5647,.T.);
#8400=EDGE_CURVE('',#6804,#6805,#5648,.T.);
#8401=EDGE_CURVE('',#6806,#6805,#5649,.T.);
#8402=EDGE_CURVE('',#6806,#6807,#5650,.T.);
#8403=EDGE_CURVE('',#6808,#6807,#5651,.T.);
#8404=EDGE_CURVE('',#6808,#6809,#5652,.T.);
#8405=EDGE_CURVE('',#6810,#6809,#5653,.T.);
#8406=EDGE_CURVE('',#6810,#6811,#5654,.T.);
#8407=EDGE_CURVE('',#6812,#6811,#5655,.T.);
#8408=EDGE_CURVE('',#6812,#6813,#5656,.T.);
#8409=EDGE_CURVE('',#6814,#6813,#5657,.T.);
#8410=EDGE_CURVE('',#6814,#6815,#5658,.T.);
#8411=EDGE_CURVE('',#6816,#6815,#5659,.T.);
#8412=EDGE_CURVE('',#6816,#6817,#5660,.T.);
#8413=EDGE_CURVE('',#6818,#6817,#5661,.T.);
#8414=EDGE_CURVE('',#6818,#6819,#5662,.T.);
#8415=EDGE_CURVE('',#6820,#6819,#5663,.T.);
#8416=EDGE_CURVE('',#6820,#6821,#5664,.T.);
#8417=EDGE_CURVE('',#6782,#6821,#5665,.T.);
#8418=EDGE_CURVE('',#6822,#6822,#5666,.T.);
#8419=EDGE_CURVE('',#6822,#6781,#4075,.T.);
#8420=EDGE_CURVE('',#6823,#6823,#5667,.T.);
#8421=EDGE_CURVE('',#6824,#6825,#5668,.T.);
#8422=EDGE_CURVE('',#6825,#6826,#5669,.T.);
#8423=EDGE_CURVE('',#6826,#6827,#5670,.T.);
#8424=EDGE_CURVE('',#6827,#6828,#5671,.T.);
#8425=EDGE_CURVE('',#6828,#6829,#5672,.T.);
#8426=EDGE_CURVE('',#6829,#6830,#5673,.T.);
#8427=EDGE_CURVE('',#6830,#6831,#5674,.T.);
#8428=EDGE_CURVE('',#6831,#6832,#5675,.T.);
#8429=EDGE_CURVE('',#6832,#6833,#5676,.T.);
#8430=EDGE_CURVE('',#6833,#6834,#5677,.T.);
#8431=EDGE_CURVE('',#6834,#6835,#5678,.T.);
#8432=EDGE_CURVE('',#6835,#6836,#5679,.T.);
#8433=EDGE_CURVE('',#6836,#6837,#5680,.T.);
#8434=EDGE_CURVE('',#6837,#6838,#5681,.T.);
#8435=EDGE_CURVE('',#6838,#6839,#5682,.T.);
#8436=EDGE_CURVE('',#6839,#6840,#5683,.T.);
#8437=EDGE_CURVE('',#6840,#6841,#5684,.T.);
#8438=EDGE_CURVE('',#6841,#6842,#5685,.T.);
#8439=EDGE_CURVE('',#6842,#6843,#5686,.T.);
#8440=EDGE_CURVE('',#6843,#6844,#5687,.T.);
#8441=EDGE_CURVE('',#6844,#6845,#5688,.T.);
#8442=EDGE_CURVE('',#6845,#6846,#5689,.T.);
#8443=EDGE_CURVE('',#6846,#6847,#5690,.T.);
#8444=EDGE_CURVE('',#6847,#6848,#5691,.T.);
#8445=EDGE_CURVE('',#6848,#6849,#5692,.T.);
#8446=EDGE_CURVE('',#6849,#6850,#5693,.T.);
#8447=EDGE_CURVE('',#6850,#6851,#5694,.T.);
#8448=EDGE_CURVE('',#6851,#6852,#5695,.T.);
#8449=EDGE_CURVE('',#6852,#6853,#5696,.T.);
#8450=EDGE_CURVE('',#6853,#6854,#5697,.T.);
#8451=EDGE_CURVE('',#6854,#6855,#5698,.T.);
#8452=EDGE_CURVE('',#6855,#6856,#5699,.T.);
#8453=EDGE_CURVE('',#6856,#6857,#5700,.T.);
#8454=EDGE_CURVE('',#6857,#6858,#5701,.T.);
#8455=EDGE_CURVE('',#6858,#6859,#5702,.T.);
#8456=EDGE_CURVE('',#6859,#6860,#5703,.T.);
#8457=EDGE_CURVE('',#6860,#6861,#5704,.T.);
#8458=EDGE_CURVE('',#6861,#6862,#5705,.T.);
#8459=EDGE_CURVE('',#6862,#6863,#5706,.T.);
#8460=EDGE_CURVE('',#6863,#6824,#5707,.T.);
#8461=EDGE_CURVE('',#6864,#6864,#5708,.T.);
#8462=EDGE_CURVE('',#6864,#6823,#4076,.T.);
#8463=EDGE_CURVE('',#6825,#6782,#4077,.T.);
#8464=EDGE_CURVE('',#6783,#6824,#4078,.T.);
#8465=EDGE_CURVE('',#6863,#6784,#4079,.T.);
#8466=EDGE_CURVE('',#6785,#6862,#4080,.T.);
#8467=EDGE_CURVE('',#6861,#6786,#4081,.T.);
#8468=EDGE_CURVE('',#6787,#6860,#4082,.T.);
#8469=EDGE_CURVE('',#6859,#6788,#4083,.T.);
#8470=EDGE_CURVE('',#6789,#6858,#4084,.T.);
#8471=EDGE_CURVE('',#6857,#6790,#4085,.T.);
#8472=EDGE_CURVE('',#6791,#6856,#4086,.T.);
#8473=EDGE_CURVE('',#6855,#6792,#4087,.T.);
#8474=EDGE_CURVE('',#6793,#6854,#4088,.T.);
#8475=EDGE_CURVE('',#6853,#6794,#4089,.T.);
#8476=EDGE_CURVE('',#6795,#6852,#4090,.T.);
#8477=EDGE_CURVE('',#6851,#6796,#4091,.T.);
#8478=EDGE_CURVE('',#6797,#6850,#4092,.T.);
#8479=EDGE_CURVE('',#6849,#6798,#4093,.T.);
#8480=EDGE_CURVE('',#6799,#6848,#4094,.T.);
#8481=EDGE_CURVE('',#6847,#6800,#4095,.T.);
#8482=EDGE_CURVE('',#6801,#6846,#4096,.T.);
#8483=EDGE_CURVE('',#6845,#6802,#4097,.T.);
#8484=EDGE_CURVE('',#6803,#6844,#4098,.T.);
#8485=EDGE_CURVE('',#6843,#6804,#4099,.T.);
#8486=EDGE_CURVE('',#6805,#6842,#4100,.T.);
#8487=EDGE_CURVE('',#6841,#6806,#4101,.T.);
#8488=EDGE_CURVE('',#6807,#6840,#4102,.T.);
#8489=EDGE_CURVE('',#6839,#6808,#4103,.T.);
#8490=EDGE_CURVE('',#6809,#6838,#4104,.T.);
#8491=EDGE_CURVE('',#6837,#6810,#4105,.T.);
#8492=EDGE_CURVE('',#6811,#6836,#4106,.T.);
#8493=EDGE_CURVE('',#6835,#6812,#4107,.T.);
#8494=EDGE_CURVE('',#6813,#6834,#4108,.T.);
#8495=EDGE_CURVE('',#6833,#6814,#4109,.T.);
#8496=EDGE_CURVE('',#6815,#6832,#4110,.T.);
#8497=EDGE_CURVE('',#6831,#6816,#4111,.T.);
#8498=EDGE_CURVE('',#6817,#6830,#4112,.T.);
#8499=EDGE_CURVE('',#6829,#6818,#4113,.T.);
#8500=EDGE_CURVE('',#6819,#6828,#4114,.T.);
#8501=EDGE_CURVE('',#6821,#6826,#4115,.T.);
#8502=EDGE_CURVE('',#6827,#6820,#4116,.T.);
#11302=ORIENTED_EDGE('',*,*,#8343,.F.);
#11303=ORIENTED_EDGE('',*,*,#8344,.F.);
#11304=ORIENTED_EDGE('',*,*,#8345,.F.);
#11305=ORIENTED_EDGE('',*,*,#8346,.T.);
#11306=ORIENTED_EDGE('',*,*,#8347,.F.);
#11307=ORIENTED_EDGE('',*,*,#8348,.F.);
#11308=ORIENTED_EDGE('',*,*,#8349,.F.);
#11309=ORIENTED_EDGE('',*,*,#8350,.F.);
#11310=ORIENTED_EDGE('',*,*,#8346,.F.);
#11311=ORIENTED_EDGE('',*,*,#8351,.F.);
#11312=ORIENTED_EDGE('',*,*,#8352,.F.);
#11313=ORIENTED_EDGE('',*,*,#8353,.T.);
#11314=ORIENTED_EDGE('',*,*,#8354,.F.);
#11315=ORIENTED_EDGE('',*,*,#8355,.F.);
#11316=ORIENTED_EDGE('',*,*,#8356,.F.);
#11317=ORIENTED_EDGE('',*,*,#8353,.F.);
#11318=ORIENTED_EDGE('',*,*,#8357,.F.);
#11319=ORIENTED_EDGE('',*,*,#8358,.T.);
#11320=ORIENTED_EDGE('',*,*,#8344,.T.);
#11321=ORIENTED_EDGE('',*,*,#8359,.T.);
#11322=ORIENTED_EDGE('',*,*,#8360,.F.);
#11323=ORIENTED_EDGE('',*,*,#8359,.F.);
#11324=ORIENTED_EDGE('',*,*,#8343,.T.);
#11325=ORIENTED_EDGE('',*,*,#8345,.T.);
#11326=ORIENTED_EDGE('',*,*,#8358,.F.);
#11327=ORIENTED_EDGE('',*,*,#8355,.T.);
#11328=ORIENTED_EDGE('',*,*,#8354,.T.);
#11329=ORIENTED_EDGE('',*,*,#8356,.T.);
#11330=ORIENTED_EDGE('',*,*,#8361,.T.);
#11331=ORIENTED_EDGE('',*,*,#8362,.T.);
#11332=ORIENTED_EDGE('',*,*,#8363,.T.);
#11333=ORIENTED_EDGE('',*,*,#8364,.T.);
#11334=ORIENTED_EDGE('',*,*,#8365,.T.);
#11335=ORIENTED_EDGE('',*,*,#8366,.T.);
#11336=ORIENTED_EDGE('',*,*,#8362,.F.);
#11337=ORIENTED_EDGE('',*,*,#8361,.F.);
#11338=ORIENTED_EDGE('',*,*,#8363,.F.);
#11339=ORIENTED_EDGE('',*,*,#8367,.T.);
#11340=ORIENTED_EDGE('',*,*,#8368,.F.);
#11341=ORIENTED_EDGE('',*,*,#8369,.F.);
#11342=ORIENTED_EDGE('',*,*,#8367,.F.);
#11343=ORIENTED_EDGE('',*,*,#8370,.F.);
#11344=ORIENTED_EDGE('',*,*,#8371,.F.);
#11345=ORIENTED_EDGE('',*,*,#8372,.T.);
#11346=ORIENTED_EDGE('',*,*,#8365,.F.);
#11347=ORIENTED_EDGE('',*,*,#8364,.F.);
#11348=ORIENTED_EDGE('',*,*,#8366,.F.);
#11349=ORIENTED_EDGE('',*,*,#8372,.F.);
#11350=ORIENTED_EDGE('',*,*,#8373,.F.);
#11351=ORIENTED_EDGE('',*,*,#8374,.T.);
#11352=ORIENTED_EDGE('',*,*,#8347,.T.);
#11353=ORIENTED_EDGE('',*,*,#8350,.T.);
#11354=ORIENTED_EDGE('',*,*,#8375,.T.);
#11355=ORIENTED_EDGE('',*,*,#8376,.F.);
#11356=ORIENTED_EDGE('',*,*,#8375,.F.);
#11357=ORIENTED_EDGE('',*,*,#8349,.T.);
#11358=ORIENTED_EDGE('',*,*,#8348,.T.);
#11359=ORIENTED_EDGE('',*,*,#8374,.F.);
#11360=ORIENTED_EDGE('',*,*,#8351,.T.);
#11361=ORIENTED_EDGE('',*,*,#8352,.T.);
#11362=ORIENTED_EDGE('',*,*,#8370,.T.);
#11363=ORIENTED_EDGE('',*,*,#8371,.T.);
#11364=ORIENTED_EDGE('',*,*,#8368,.T.);
#11365=ORIENTED_EDGE('',*,*,#8369,.T.);
#11366=ORIENTED_EDGE('',*,*,#8357,.T.);
#11367=ORIENTED_EDGE('',*,*,#8373,.T.);
#11368=ORIENTED_EDGE('',*,*,#8377,.T.);
#11369=ORIENTED_EDGE('',*,*,#8378,.T.);
#11370=ORIENTED_EDGE('',*,*,#8379,.F.);
#11371=ORIENTED_EDGE('',*,*,#8380,.T.);
#11372=ORIENTED_EDGE('',*,*,#8381,.F.);
#11373=ORIENTED_EDGE('',*,*,#8382,.T.);
#11374=ORIENTED_EDGE('',*,*,#8383,.F.);
#11375=ORIENTED_EDGE('',*,*,#8384,.T.);
#11376=ORIENTED_EDGE('',*,*,#8385,.F.);
#11377=ORIENTED_EDGE('',*,*,#8386,.T.);
#11378=ORIENTED_EDGE('',*,*,#8387,.F.);
#11379=ORIENTED_EDGE('',*,*,#8388,.T.);
#11380=ORIENTED_EDGE('',*,*,#8389,.F.);
#11381=ORIENTED_EDGE('',*,*,#8390,.T.);
#11382=ORIENTED_EDGE('',*,*,#8391,.F.);
#11383=ORIENTED_EDGE('',*,*,#8392,.T.);
#11384=ORIENTED_EDGE('',*,*,#8393,.F.);
#11385=ORIENTED_EDGE('',*,*,#8394,.T.);
#11386=ORIENTED_EDGE('',*,*,#8395,.F.);
#11387=ORIENTED_EDGE('',*,*,#8396,.T.);
#11388=ORIENTED_EDGE('',*,*,#8397,.F.);
#11389=ORIENTED_EDGE('',*,*,#8398,.T.);
#11390=ORIENTED_EDGE('',*,*,#8399,.F.);
#11391=ORIENTED_EDGE('',*,*,#8400,.T.);
#11392=ORIENTED_EDGE('',*,*,#8401,.F.);
#11393=ORIENTED_EDGE('',*,*,#8402,.T.);
#11394=ORIENTED_EDGE('',*,*,#8403,.F.);
#11395=ORIENTED_EDGE('',*,*,#8404,.T.);
#11396=ORIENTED_EDGE('',*,*,#8405,.F.);
#11397=ORIENTED_EDGE('',*,*,#8406,.T.);
#11398=ORIENTED_EDGE('',*,*,#8407,.F.);
#11399=ORIENTED_EDGE('',*,*,#8408,.T.);
#11400=ORIENTED_EDGE('',*,*,#8409,.F.);
#11401=ORIENTED_EDGE('',*,*,#8410,.T.);
#11402=ORIENTED_EDGE('',*,*,#8411,.F.);
#11403=ORIENTED_EDGE('',*,*,#8412,.T.);
#11404=ORIENTED_EDGE('',*,*,#8413,.F.);
#11405=ORIENTED_EDGE('',*,*,#8414,.T.);
#11406=ORIENTED_EDGE('',*,*,#8415,.F.);
#11407=ORIENTED_EDGE('',*,*,#8416,.T.);
#11408=ORIENTED_EDGE('',*,*,#8417,.F.);
#11409=ORIENTED_EDGE('',*,*,#8418,.F.);
#11410=ORIENTED_EDGE('',*,*,#8419,.T.);
#11411=ORIENTED_EDGE('',*,*,#8377,.F.);
#11412=ORIENTED_EDGE('',*,*,#8419,.F.);
#11413=ORIENTED_EDGE('',*,*,#8418,.T.);
#11414=ORIENTED_EDGE('',*,*,#8360,.T.);
#11415=ORIENTED_EDGE('',*,*,#8420,.F.);
#11416=ORIENTED_EDGE('',*,*,#8421,.T.);
#11417=ORIENTED_EDGE('',*,*,#8422,.T.);
#11418=ORIENTED_EDGE('',*,*,#8423,.T.);
#11419=ORIENTED_EDGE('',*,*,#8424,.T.);
#11420=ORIENTED_EDGE('',*,*,#8425,.T.);
#11421=ORIENTED_EDGE('',*,*,#8426,.T.);
#11422=ORIENTED_EDGE('',*,*,#8427,.T.);
#11423=ORIENTED_EDGE('',*,*,#8428,.T.);
#11424=ORIENTED_EDGE('',*,*,#8429,.T.);
#11425=ORIENTED_EDGE('',*,*,#8430,.T.);
#11426=ORIENTED_EDGE('',*,*,#8431,.T.);
#11427=ORIENTED_EDGE('',*,*,#8432,.T.);
#11428=ORIENTED_EDGE('',*,*,#8433,.T.);
#11429=ORIENTED_EDGE('',*,*,#8434,.T.);
#11430=ORIENTED_EDGE('',*,*,#8435,.T.);
#11431=ORIENTED_EDGE('',*,*,#8436,.T.);
#11432=ORIENTED_EDGE('',*,*,#8437,.T.);
#11433=ORIENTED_EDGE('',*,*,#8438,.T.);
#11434=ORIENTED_EDGE('',*,*,#8439,.T.);
#11435=ORIENTED_EDGE('',*,*,#8440,.T.);
#11436=ORIENTED_EDGE('',*,*,#8441,.T.);
#11437=ORIENTED_EDGE('',*,*,#8442,.T.);
#11438=ORIENTED_EDGE('',*,*,#8443,.T.);
#11439=ORIENTED_EDGE('',*,*,#8444,.T.);
#11440=ORIENTED_EDGE('',*,*,#8445,.T.);
#11441=ORIENTED_EDGE('',*,*,#8446,.T.);
#11442=ORIENTED_EDGE('',*,*,#8447,.T.);
#11443=ORIENTED_EDGE('',*,*,#8448,.T.);
#11444=ORIENTED_EDGE('',*,*,#8449,.T.);
#11445=ORIENTED_EDGE('',*,*,#8450,.T.);
#11446=ORIENTED_EDGE('',*,*,#8451,.T.);
#11447=ORIENTED_EDGE('',*,*,#8452,.T.);
#11448=ORIENTED_EDGE('',*,*,#8453,.T.);
#11449=ORIENTED_EDGE('',*,*,#8454,.T.);
#11450=ORIENTED_EDGE('',*,*,#8455,.T.);
#11451=ORIENTED_EDGE('',*,*,#8456,.T.);
#11452=ORIENTED_EDGE('',*,*,#8457,.T.);
#11453=ORIENTED_EDGE('',*,*,#8458,.T.);
#11454=ORIENTED_EDGE('',*,*,#8459,.T.);
#11455=ORIENTED_EDGE('',*,*,#8460,.T.);
#11456=ORIENTED_EDGE('',*,*,#8461,.F.);
#11457=ORIENTED_EDGE('',*,*,#8462,.T.);
#11458=ORIENTED_EDGE('',*,*,#8420,.T.);
#11459=ORIENTED_EDGE('',*,*,#8462,.F.);
#11460=ORIENTED_EDGE('',*,*,#8461,.T.);
#11461=ORIENTED_EDGE('',*,*,#8376,.T.);
#11462=ORIENTED_EDGE('',*,*,#8463,.F.);
#11463=ORIENTED_EDGE('',*,*,#8421,.F.);
#11464=ORIENTED_EDGE('',*,*,#8464,.F.);
#11465=ORIENTED_EDGE('',*,*,#8378,.F.);
#11466=ORIENTED_EDGE('',*,*,#8464,.T.);
#11467=ORIENTED_EDGE('',*,*,#8460,.F.);
#11468=ORIENTED_EDGE('',*,*,#8465,.T.);
#11469=ORIENTED_EDGE('',*,*,#8379,.T.);
#11470=ORIENTED_EDGE('',*,*,#8465,.F.);
#11471=ORIENTED_EDGE('',*,*,#8459,.F.);
#11472=ORIENTED_EDGE('',*,*,#8466,.F.);
#11473=ORIENTED_EDGE('',*,*,#8380,.F.);
#11474=ORIENTED_EDGE('',*,*,#8466,.T.);
#11475=ORIENTED_EDGE('',*,*,#8458,.F.);
#11476=ORIENTED_EDGE('',*,*,#8467,.T.);
#11477=ORIENTED_EDGE('',*,*,#8381,.T.);
#11478=ORIENTED_EDGE('',*,*,#8467,.F.);
#11479=ORIENTED_EDGE('',*,*,#8457,.F.);
#11480=ORIENTED_EDGE('',*,*,#8468,.F.);
#11481=ORIENTED_EDGE('',*,*,#8382,.F.);
#11482=ORIENTED_EDGE('',*,*,#8468,.T.);
#11483=ORIENTED_EDGE('',*,*,#8456,.F.);
#11484=ORIENTED_EDGE('',*,*,#8469,.T.);
#11485=ORIENTED_EDGE('',*,*,#8383,.T.);
#11486=ORIENTED_EDGE('',*,*,#8469,.F.);
#11487=ORIENTED_EDGE('',*,*,#8455,.F.);
#11488=ORIENTED_EDGE('',*,*,#8470,.F.);
#11489=ORIENTED_EDGE('',*,*,#8384,.F.);
#11490=ORIENTED_EDGE('',*,*,#8470,.T.);
#11491=ORIENTED_EDGE('',*,*,#8454,.F.);
#11492=ORIENTED_EDGE('',*,*,#8471,.T.);
#11493=ORIENTED_EDGE('',*,*,#8385,.T.);
#11494=ORIENTED_EDGE('',*,*,#8471,.F.);
#11495=ORIENTED_EDGE('',*,*,#8453,.F.);
#11496=ORIENTED_EDGE('',*,*,#8472,.F.);
#11497=ORIENTED_EDGE('',*,*,#8386,.F.);
#11498=ORIENTED_EDGE('',*,*,#8472,.T.);
#11499=ORIENTED_EDGE('',*,*,#8452,.F.);
#11500=ORIENTED_EDGE('',*,*,#8473,.T.);
#11501=ORIENTED_EDGE('',*,*,#8387,.T.);
#11502=ORIENTED_EDGE('',*,*,#8473,.F.);
#11503=ORIENTED_EDGE('',*,*,#8451,.F.);
#11504=ORIENTED_EDGE('',*,*,#8474,.F.);
#11505=ORIENTED_EDGE('',*,*,#8388,.F.);
#11506=ORIENTED_EDGE('',*,*,#8474,.T.);
#11507=ORIENTED_EDGE('',*,*,#8450,.F.);
#11508=ORIENTED_EDGE('',*,*,#8475,.T.);
#11509=ORIENTED_EDGE('',*,*,#8389,.T.);
#11510=ORIENTED_EDGE('',*,*,#8475,.F.);
#11511=ORIENTED_EDGE('',*,*,#8449,.F.);
#11512=ORIENTED_EDGE('',*,*,#8476,.F.);
#11513=ORIENTED_EDGE('',*,*,#8390,.F.);
#11514=ORIENTED_EDGE('',*,*,#8476,.T.);
#11515=ORIENTED_EDGE('',*,*,#8448,.F.);
#11516=ORIENTED_EDGE('',*,*,#8477,.T.);
#11517=ORIENTED_EDGE('',*,*,#8391,.T.);
#11518=ORIENTED_EDGE('',*,*,#8477,.F.);
#11519=ORIENTED_EDGE('',*,*,#8447,.F.);
#11520=ORIENTED_EDGE('',*,*,#8478,.F.);
#11521=ORIENTED_EDGE('',*,*,#8392,.F.);
#11522=ORIENTED_EDGE('',*,*,#8478,.T.);
#11523=ORIENTED_EDGE('',*,*,#8446,.F.);
#11524=ORIENTED_EDGE('',*,*,#8479,.T.);
#11525=ORIENTED_EDGE('',*,*,#8393,.T.);
#11526=ORIENTED_EDGE('',*,*,#8479,.F.);
#11527=ORIENTED_EDGE('',*,*,#8445,.F.);
#11528=ORIENTED_EDGE('',*,*,#8480,.F.);
#11529=ORIENTED_EDGE('',*,*,#8394,.F.);
#11530=ORIENTED_EDGE('',*,*,#8480,.T.);
#11531=ORIENTED_EDGE('',*,*,#8444,.F.);
#11532=ORIENTED_EDGE('',*,*,#8481,.T.);
#11533=ORIENTED_EDGE('',*,*,#8395,.T.);
#11534=ORIENTED_EDGE('',*,*,#8481,.F.);
#11535=ORIENTED_EDGE('',*,*,#8443,.F.);
#11536=ORIENTED_EDGE('',*,*,#8482,.F.);
#11537=ORIENTED_EDGE('',*,*,#8396,.F.);
#11538=ORIENTED_EDGE('',*,*,#8482,.T.);
#11539=ORIENTED_EDGE('',*,*,#8442,.F.);
#11540=ORIENTED_EDGE('',*,*,#8483,.T.);
#11541=ORIENTED_EDGE('',*,*,#8397,.T.);
#11542=ORIENTED_EDGE('',*,*,#8483,.F.);
#11543=ORIENTED_EDGE('',*,*,#8441,.F.);
#11544=ORIENTED_EDGE('',*,*,#8484,.F.);
#11545=ORIENTED_EDGE('',*,*,#8398,.F.);
#11546=ORIENTED_EDGE('',*,*,#8484,.T.);
#11547=ORIENTED_EDGE('',*,*,#8440,.F.);
#11548=ORIENTED_EDGE('',*,*,#8485,.T.);
#11549=ORIENTED_EDGE('',*,*,#8399,.T.);
#11550=ORIENTED_EDGE('',*,*,#8485,.F.);
#11551=ORIENTED_EDGE('',*,*,#8439,.F.);
#11552=ORIENTED_EDGE('',*,*,#8486,.F.);
#11553=ORIENTED_EDGE('',*,*,#8400,.F.);
#11554=ORIENTED_EDGE('',*,*,#8486,.T.);
#11555=ORIENTED_EDGE('',*,*,#8438,.F.);
#11556=ORIENTED_EDGE('',*,*,#8487,.T.);
#11557=ORIENTED_EDGE('',*,*,#8401,.T.);
#11558=ORIENTED_EDGE('',*,*,#8487,.F.);
#11559=ORIENTED_EDGE('',*,*,#8437,.F.);
#11560=ORIENTED_EDGE('',*,*,#8488,.F.);
#11561=ORIENTED_EDGE('',*,*,#8402,.F.);
#11562=ORIENTED_EDGE('',*,*,#8488,.T.);
#11563=ORIENTED_EDGE('',*,*,#8436,.F.);
#11564=ORIENTED_EDGE('',*,*,#8489,.T.);
#11565=ORIENTED_EDGE('',*,*,#8403,.T.);
#11566=ORIENTED_EDGE('',*,*,#8489,.F.);
#11567=ORIENTED_EDGE('',*,*,#8435,.F.);
#11568=ORIENTED_EDGE('',*,*,#8490,.F.);
#11569=ORIENTED_EDGE('',*,*,#8404,.F.);
#11570=ORIENTED_EDGE('',*,*,#8490,.T.);
#11571=ORIENTED_EDGE('',*,*,#8434,.F.);
#11572=ORIENTED_EDGE('',*,*,#8491,.T.);
#11573=ORIENTED_EDGE('',*,*,#8405,.T.);
#11574=ORIENTED_EDGE('',*,*,#8491,.F.);
#11575=ORIENTED_EDGE('',*,*,#8433,.F.);
#11576=ORIENTED_EDGE('',*,*,#8492,.F.);
#11577=ORIENTED_EDGE('',*,*,#8406,.F.);
#11578=ORIENTED_EDGE('',*,*,#8492,.T.);
#11579=ORIENTED_EDGE('',*,*,#8432,.F.);
#11580=ORIENTED_EDGE('',*,*,#8493,.T.);
#11581=ORIENTED_EDGE('',*,*,#8407,.T.);
#11582=ORIENTED_EDGE('',*,*,#8493,.F.);
#11583=ORIENTED_EDGE('',*,*,#8431,.F.);
#11584=ORIENTED_EDGE('',*,*,#8494,.F.);
#11585=ORIENTED_EDGE('',*,*,#8408,.F.);
#11586=ORIENTED_EDGE('',*,*,#8494,.T.);
#11587=ORIENTED_EDGE('',*,*,#8430,.F.);
#11588=ORIENTED_EDGE('',*,*,#8495,.T.);
#11589=ORIENTED_EDGE('',*,*,#8409,.T.);
#11590=ORIENTED_EDGE('',*,*,#8495,.F.);
#11591=ORIENTED_EDGE('',*,*,#8429,.F.);
#11592=ORIENTED_EDGE('',*,*,#8496,.F.);
#11593=ORIENTED_EDGE('',*,*,#8410,.F.);
#11594=ORIENTED_EDGE('',*,*,#8496,.T.);
#11595=ORIENTED_EDGE('',*,*,#8428,.F.);
#11596=ORIENTED_EDGE('',*,*,#8497,.T.);
#11597=ORIENTED_EDGE('',*,*,#8411,.T.);
#11598=ORIENTED_EDGE('',*,*,#8497,.F.);
#11599=ORIENTED_EDGE('',*,*,#8427,.F.);
#11600=ORIENTED_EDGE('',*,*,#8498,.F.);
#11601=ORIENTED_EDGE('',*,*,#8412,.F.);
#11602=ORIENTED_EDGE('',*,*,#8498,.T.);
#11603=ORIENTED_EDGE('',*,*,#8426,.F.);
#11604=ORIENTED_EDGE('',*,*,#8499,.T.);
#11605=ORIENTED_EDGE('',*,*,#8413,.T.);
#11606=ORIENTED_EDGE('',*,*,#8500,.F.);
#11607=ORIENTED_EDGE('',*,*,#8414,.F.);
#11608=ORIENTED_EDGE('',*,*,#8499,.F.);
#11609=ORIENTED_EDGE('',*,*,#8425,.F.);
#11610=ORIENTED_EDGE('',*,*,#8463,.T.);
#11611=ORIENTED_EDGE('',*,*,#8417,.T.);
#11612=ORIENTED_EDGE('',*,*,#8501,.T.);
#11613=ORIENTED_EDGE('',*,*,#8422,.F.);
#11614=ORIENTED_EDGE('',*,*,#8502,.F.);
#11615=ORIENTED_EDGE('',*,*,#8423,.F.);
#11616=ORIENTED_EDGE('',*,*,#8501,.F.);
#11617=ORIENTED_EDGE('',*,*,#8416,.F.);
#11618=ORIENTED_EDGE('',*,*,#8500,.T.);
#11619=ORIENTED_EDGE('',*,*,#8424,.F.);
#11620=ORIENTED_EDGE('',*,*,#8502,.T.);
#11621=ORIENTED_EDGE('',*,*,#8415,.T.);
#12743=CYLINDRICAL_SURFACE('',#15730,0.125);
#12744=CYLINDRICAL_SURFACE('',#15731,0.125);
#12745=CYLINDRICAL_SURFACE('',#15732,0.65);
#12746=CYLINDRICAL_SURFACE('',#15735,0.125);
#12747=CYLINDRICAL_SURFACE('',#15736,0.125);
#12748=CYLINDRICAL_SURFACE('',#15737,0.4);
#12749=CYLINDRICAL_SURFACE('',#15783,0.8);
#12750=CYLINDRICAL_SURFACE('',#15828,0.8);
#12751=CYLINDRICAL_SURFACE('',#15831,0.0555);
#12752=CYLINDRICAL_SURFACE('',#15832,0.611219772367581);
#12753=CYLINDRICAL_SURFACE('',#15833,0.0555);
#12754=CYLINDRICAL_SURFACE('',#15834,0.611219772367581);
#12755=CYLINDRICAL_SURFACE('',#15835,0.0555);
#12756=CYLINDRICAL_SURFACE('',#15836,0.611219772367581);
#12757=CYLINDRICAL_SURFACE('',#15837,0.0555);
#12758=CYLINDRICAL_SURFACE('',#15838,0.611219772367581);
#12759=CYLINDRICAL_SURFACE('',#15839,0.0555);
#12760=CYLINDRICAL_SURFACE('',#15840,0.611219772367581);
#12761=CYLINDRICAL_SURFACE('',#15841,0.0555);
#12762=CYLINDRICAL_SURFACE('',#15842,0.611219772367581);
#12763=CYLINDRICAL_SURFACE('',#15843,0.0555);
#12764=CYLINDRICAL_SURFACE('',#15844,0.611219772367581);
#12765=CYLINDRICAL_SURFACE('',#15845,0.0555);
#12766=CYLINDRICAL_SURFACE('',#15846,0.611219772367581);
#12767=CYLINDRICAL_SURFACE('',#15847,0.0555);
#12768=CYLINDRICAL_SURFACE('',#15848,0.611219772367581);
#12769=CYLINDRICAL_SURFACE('',#15849,0.0555);
#12770=CYLINDRICAL_SURFACE('',#15850,0.611219772367581);
#12771=CYLINDRICAL_SURFACE('',#15851,0.0555);
#12772=CYLINDRICAL_SURFACE('',#15852,0.611219772367581);
#12773=CYLINDRICAL_SURFACE('',#15853,0.0555);
#12774=CYLINDRICAL_SURFACE('',#15854,0.611219772367581);
#12775=CYLINDRICAL_SURFACE('',#15855,0.0555);
#12776=CYLINDRICAL_SURFACE('',#15856,0.611219772367581);
#12777=CYLINDRICAL_SURFACE('',#15857,0.0555);
#12778=CYLINDRICAL_SURFACE('',#15858,0.611219772367581);
#12779=CYLINDRICAL_SURFACE('',#15859,0.0555);
#12780=CYLINDRICAL_SURFACE('',#15860,0.611219772367581);
#12781=CYLINDRICAL_SURFACE('',#15861,0.0555);
#12782=CYLINDRICAL_SURFACE('',#15862,0.611219772367581);
#12783=CYLINDRICAL_SURFACE('',#15863,0.0555);
#12784=CYLINDRICAL_SURFACE('',#15864,0.611219772367581);
#12785=CYLINDRICAL_SURFACE('',#15865,0.0555);
#12786=CYLINDRICAL_SURFACE('',#15866,0.611219772367581);
#12787=CYLINDRICAL_SURFACE('',#15867,0.0555);
#12788=CYLINDRICAL_SURFACE('',#15868,0.611219772367581);
#12789=CYLINDRICAL_SURFACE('',#15869,0.0555);
#12790=CYLINDRICAL_SURFACE('',#15870,0.611219772367581);
#13470=ADVANCED_FACE('',(#2191),#12743,.F.);
#13471=ADVANCED_FACE('',(#2192),#12744,.F.);
#13472=ADVANCED_FACE('',(#2193,#1222,#1223,#1224),#12745,.T.);
#13473=ADVANCED_FACE('',(#2194),#12746,.F.);
#13474=ADVANCED_FACE('',(#2195),#12747,.F.);
#13475=ADVANCED_FACE('',(#2196,#1225,#1226,#1227),#12748,.F.);
#13476=ADVANCED_FACE('',(#2197,#1228),#1566,.F.);
#13477=ADVANCED_FACE('',(#2198,#1229),#1567,.T.);
#13478=ADVANCED_FACE('',(#2199),#12749,.T.);
#13479=ADVANCED_FACE('',(#2200,#1230),#1568,.F.);
#13480=ADVANCED_FACE('',(#2201,#1231),#1569,.F.);
#13481=ADVANCED_FACE('',(#2202),#12750,.T.);
#13482=ADVANCED_FACE('',(#2203,#1232),#1570,.T.);
#13483=ADVANCED_FACE('',(#2204),#12751,.F.);
#13484=ADVANCED_FACE('',(#2205),#12752,.T.);
#13485=ADVANCED_FACE('',(#2206),#12753,.F.);
#13486=ADVANCED_FACE('',(#2207),#12754,.T.);
#13487=ADVANCED_FACE('',(#2208),#12755,.F.);
#13488=ADVANCED_FACE('',(#2209),#12756,.T.);
#13489=ADVANCED_FACE('',(#2210),#12757,.F.);
#13490=ADVANCED_FACE('',(#2211),#12758,.T.);
#13491=ADVANCED_FACE('',(#2212),#12759,.F.);
#13492=ADVANCED_FACE('',(#2213),#12760,.T.);
#13493=ADVANCED_FACE('',(#2214),#12761,.F.);
#13494=ADVANCED_FACE('',(#2215),#12762,.T.);
#13495=ADVANCED_FACE('',(#2216),#12763,.F.);
#13496=ADVANCED_FACE('',(#2217),#12764,.T.);
#13497=ADVANCED_FACE('',(#2218),#12765,.F.);
#13498=ADVANCED_FACE('',(#2219),#12766,.T.);
#13499=ADVANCED_FACE('',(#2220),#12767,.F.);
#13500=ADVANCED_FACE('',(#2221),#12768,.T.);
#13501=ADVANCED_FACE('',(#2222),#12769,.F.);
#13502=ADVANCED_FACE('',(#2223),#12770,.T.);
#13503=ADVANCED_FACE('',(#2224),#12771,.F.);
#13504=ADVANCED_FACE('',(#2225),#12772,.T.);
#13505=ADVANCED_FACE('',(#2226),#12773,.F.);
#13506=ADVANCED_FACE('',(#2227),#12774,.T.);
#13507=ADVANCED_FACE('',(#2228),#12775,.F.);
#13508=ADVANCED_FACE('',(#2229),#12776,.T.);
#13509=ADVANCED_FACE('',(#2230),#12777,.F.);
#13510=ADVANCED_FACE('',(#2231),#12778,.T.);
#13511=ADVANCED_FACE('',(#2232),#12779,.F.);
#13512=ADVANCED_FACE('',(#2233),#12780,.T.);
#13513=ADVANCED_FACE('',(#2234),#12781,.F.);
#13514=ADVANCED_FACE('',(#2235),#12782,.T.);
#13515=ADVANCED_FACE('',(#2236),#12783,.F.);
#13516=ADVANCED_FACE('',(#2237),#12784,.T.);
#13517=ADVANCED_FACE('',(#2238),#12785,.F.);
#13518=ADVANCED_FACE('',(#2239),#12786,.T.);
#13519=ADVANCED_FACE('',(#2240),#12787,.F.);
#13520=ADVANCED_FACE('',(#2241),#12788,.T.);
#13521=ADVANCED_FACE('',(#2242),#12789,.F.);
#13522=ADVANCED_FACE('',(#2243),#12790,.T.);
#13784=CLOSED_SHELL('',(#13470,#13471,#13472,#13473,#13474,#13475,#13476,
#13477,#13478,#13479,#13480,#13481,#13482,#13483,#13484,#13485,#13486,#13487,
#13488,#13489,#13490,#13491,#13492,#13493,#13494,#13495,#13496,#13497,#13498,
#13499,#13500,#13501,#13502,#13503,#13504,#13505,#13506,#13507,#13508,#13509,
#13510,#13511,#13512,#13513,#13514,#13515,#13516,#13517,#13518,#13519,#13520,
#13521,#13522));
#15729=AXIS2_PLACEMENT_3D('',#24716,#19337,#19338);
#15730=AXIS2_PLACEMENT_3D('',#24717,#19339,#19340);
#15731=AXIS2_PLACEMENT_3D('',#24804,#19342,#19343);
#15732=AXIS2_PLACEMENT_3D('',#24885,#19345,#19346);
#15733=AXIS2_PLACEMENT_3D('',#24887,#19347,#19348);
#15734=AXIS2_PLACEMENT_3D('',#24891,#19351,#19352);
#15735=AXIS2_PLACEMENT_3D('',#24974,#19353,#19354);
#15736=AXIS2_PLACEMENT_3D('',#25014,#19356,#19357);
#15737=AXIS2_PLACEMENT_3D('',#25054,#19359,#19360);
#15738=AXIS2_PLACEMENT_3D('',#25056,#19361,#19362);
#15739=AXIS2_PLACEMENT_3D('',#25060,#19365,#19366);
#15740=AXIS2_PLACEMENT_3D('',#25061,#19367,#19368);
#15741=AXIS2_PLACEMENT_3D('',#25062,#19369,#19370);
#15742=AXIS2_PLACEMENT_3D('',#25064,#19371,#19372);
#15743=AXIS2_PLACEMENT_3D('',#25067,#19373,#19374);
#15744=AXIS2_PLACEMENT_3D('',#25069,#19375,#19376);
#15745=AXIS2_PLACEMENT_3D('',#25071,#19377,#19378);
#15746=AXIS2_PLACEMENT_3D('',#25073,#19379,#19380);
#15747=AXIS2_PLACEMENT_3D('',#25075,#19381,#19382);
#15748=AXIS2_PLACEMENT_3D('',#25077,#19383,#19384);
#15749=AXIS2_PLACEMENT_3D('',#25079,#19385,#19386);
#15750=AXIS2_PLACEMENT_3D('',#25081,#19387,#19388);
#15751=AXIS2_PLACEMENT_3D('',#25083,#19389,#19390);
#15752=AXIS2_PLACEMENT_3D('',#25085,#19391,#19392);
#15753=AXIS2_PLACEMENT_3D('',#25087,#19393,#19394);
#15754=AXIS2_PLACEMENT_3D('',#25089,#19395,#19396);
#15755=AXIS2_PLACEMENT_3D('',#25091,#19397,#19398);
#15756=AXIS2_PLACEMENT_3D('',#25093,#19399,#19400);
#15757=AXIS2_PLACEMENT_3D('',#25095,#19401,#19402);
#15758=AXIS2_PLACEMENT_3D('',#25097,#19403,#19404);
#15759=AXIS2_PLACEMENT_3D('',#25099,#19405,#19406);
#15760=AXIS2_PLACEMENT_3D('',#25101,#19407,#19408);
#15761=AXIS2_PLACEMENT_3D('',#25103,#19409,#19410);
#15762=AXIS2_PLACEMENT_3D('',#25105,#19411,#19412);
#15763=AXIS2_PLACEMENT_3D('',#25107,#19413,#19414);
#15764=AXIS2_PLACEMENT_3D('',#25109,#19415,#19416);
#15765=AXIS2_PLACEMENT_3D('',#25111,#19417,#19418);
#15766=AXIS2_PLACEMENT_3D('',#25113,#19419,#19420);
#15767=AXIS2_PLACEMENT_3D('',#25115,#19421,#19422);
#15768=AXIS2_PLACEMENT_3D('',#25117,#19423,#19424);
#15769=AXIS2_PLACEMENT_3D('',#25119,#19425,#19426);
#15770=AXIS2_PLACEMENT_3D('',#25121,#19427,#19428);
#15771=AXIS2_PLACEMENT_3D('',#25123,#19429,#19430);
#15772=AXIS2_PLACEMENT_3D('',#25125,#19431,#19432);
#15773=AXIS2_PLACEMENT_3D('',#25127,#19433,#19434);
#15774=AXIS2_PLACEMENT_3D('',#25129,#19435,#19436);
#15775=AXIS2_PLACEMENT_3D('',#25131,#19437,#19438);
#15776=AXIS2_PLACEMENT_3D('',#25133,#19439,#19440);
#15777=AXIS2_PLACEMENT_3D('',#25135,#19441,#19442);
#15778=AXIS2_PLACEMENT_3D('',#25137,#19443,#19444);
#15779=AXIS2_PLACEMENT_3D('',#25139,#19445,#19446);
#15780=AXIS2_PLACEMENT_3D('',#25141,#19447,#19448);
#15781=AXIS2_PLACEMENT_3D('',#25143,#19449,#19450);
#15782=AXIS2_PLACEMENT_3D('',#25144,#19451,#19452);
#15783=AXIS2_PLACEMENT_3D('',#25145,#19453,#19454);
#15784=AXIS2_PLACEMENT_3D('',#25147,#19455,#19456);
#15785=AXIS2_PLACEMENT_3D('',#25149,#19458,#19459);
#15786=AXIS2_PLACEMENT_3D('',#25150,#19460,#19461);
#15787=AXIS2_PLACEMENT_3D('',#25152,#19462,#19463);
#15788=AXIS2_PLACEMENT_3D('',#25155,#19464,#19465);
#15789=AXIS2_PLACEMENT_3D('',#25157,#19466,#19467);
#15790=AXIS2_PLACEMENT_3D('',#25159,#19468,#19469);
#15791=AXIS2_PLACEMENT_3D('',#25161,#19470,#19471);
#15792=AXIS2_PLACEMENT_3D('',#25163,#19472,#19473);
#15793=AXIS2_PLACEMENT_3D('',#25165,#19474,#19475);
#15794=AXIS2_PLACEMENT_3D('',#25167,#19476,#19477);
#15795=AXIS2_PLACEMENT_3D('',#25169,#19478,#19479);
#15796=AXIS2_PLACEMENT_3D('',#25171,#19480,#19481);
#15797=AXIS2_PLACEMENT_3D('',#25173,#19482,#19483);
#15798=AXIS2_PLACEMENT_3D('',#25175,#19484,#19485);
#15799=AXIS2_PLACEMENT_3D('',#25177,#19486,#19487);
#15800=AXIS2_PLACEMENT_3D('',#25179,#19488,#19489);
#15801=AXIS2_PLACEMENT_3D('',#25181,#19490,#19491);
#15802=AXIS2_PLACEMENT_3D('',#25183,#19492,#19493);
#15803=AXIS2_PLACEMENT_3D('',#25185,#19494,#19495);
#15804=AXIS2_PLACEMENT_3D('',#25187,#19496,#19497);
#15805=AXIS2_PLACEMENT_3D('',#25189,#19498,#19499);
#15806=AXIS2_PLACEMENT_3D('',#25191,#19500,#19501);
#15807=AXIS2_PLACEMENT_3D('',#25193,#19502,#19503);
#15808=AXIS2_PLACEMENT_3D('',#25195,#19504,#19505);
#15809=AXIS2_PLACEMENT_3D('',#25197,#19506,#19507);
#15810=AXIS2_PLACEMENT_3D('',#25199,#19508,#19509);
#15811=AXIS2_PLACEMENT_3D('',#25201,#19510,#19511);
#15812=AXIS2_PLACEMENT_3D('',#25203,#19512,#19513);
#15813=AXIS2_PLACEMENT_3D('',#25205,#19514,#19515);
#15814=AXIS2_PLACEMENT_3D('',#25207,#19516,#19517);
#15815=AXIS2_PLACEMENT_3D('',#25209,#19518,#19519);
#15816=AXIS2_PLACEMENT_3D('',#25211,#19520,#19521);
#15817=AXIS2_PLACEMENT_3D('',#25213,#19522,#19523);
#15818=AXIS2_PLACEMENT_3D('',#25215,#19524,#19525);
#15819=AXIS2_PLACEMENT_3D('',#25217,#19526,#19527);
#15820=AXIS2_PLACEMENT_3D('',#25219,#19528,#19529);
#15821=AXIS2_PLACEMENT_3D('',#25221,#19530,#19531);
#15822=AXIS2_PLACEMENT_3D('',#25223,#19532,#19533);
#15823=AXIS2_PLACEMENT_3D('',#25225,#19534,#19535);
#15824=AXIS2_PLACEMENT_3D('',#25227,#19536,#19537);
#15825=AXIS2_PLACEMENT_3D('',#25229,#19538,#19539);
#15826=AXIS2_PLACEMENT_3D('',#25231,#19540,#19541);
#15827=AXIS2_PLACEMENT_3D('',#25232,#19542,#19543);
#15828=AXIS2_PLACEMENT_3D('',#25233,#19544,#19545);
#15829=AXIS2_PLACEMENT_3D('',#25235,#19546,#19547);
#15830=AXIS2_PLACEMENT_3D('',#25237,#19549,#19550);
#15831=AXIS2_PLACEMENT_3D('',#25238,#19551,#19552);
#15832=AXIS2_PLACEMENT_3D('',#25241,#19555,#19556);
#15833=AXIS2_PLACEMENT_3D('',#25243,#19558,#19559);
#15834=AXIS2_PLACEMENT_3D('',#25245,#19561,#19562);
#15835=AXIS2_PLACEMENT_3D('',#25247,#19564,#19565);
#15836=AXIS2_PLACEMENT_3D('',#25249,#19567,#19568);
#15837=AXIS2_PLACEMENT_3D('',#25251,#19570,#19571);
#15838=AXIS2_PLACEMENT_3D('',#25253,#19573,#19574);
#15839=AXIS2_PLACEMENT_3D('',#25255,#19576,#19577);
#15840=AXIS2_PLACEMENT_3D('',#25257,#19579,#19580);
#15841=AXIS2_PLACEMENT_3D('',#25259,#19582,#19583);
#15842=AXIS2_PLACEMENT_3D('',#25261,#19585,#19586);
#15843=AXIS2_PLACEMENT_3D('',#25263,#19588,#19589);
#15844=AXIS2_PLACEMENT_3D('',#25265,#19591,#19592);
#15845=AXIS2_PLACEMENT_3D('',#25267,#19594,#19595);
#15846=AXIS2_PLACEMENT_3D('',#25269,#19597,#19598);
#15847=AXIS2_PLACEMENT_3D('',#25271,#19600,#19601);
#15848=AXIS2_PLACEMENT_3D('',#25273,#19603,#19604);
#15849=AXIS2_PLACEMENT_3D('',#25275,#19606,#19607);
#15850=AXIS2_PLACEMENT_3D('',#25277,#19609,#19610);
#15851=AXIS2_PLACEMENT_3D('',#25279,#19612,#19613);
#15852=AXIS2_PLACEMENT_3D('',#25281,#19615,#19616);
#15853=AXIS2_PLACEMENT_3D('',#25283,#19618,#19619);
#15854=AXIS2_PLACEMENT_3D('',#25285,#19621,#19622);
#15855=AXIS2_PLACEMENT_3D('',#25287,#19624,#19625);
#15856=AXIS2_PLACEMENT_3D('',#25289,#19627,#19628);
#15857=AXIS2_PLACEMENT_3D('',#25291,#19630,#19631);
#15858=AXIS2_PLACEMENT_3D('',#25293,#19633,#19634);
#15859=AXIS2_PLACEMENT_3D('',#25295,#19636,#19637);
#15860=AXIS2_PLACEMENT_3D('',#25297,#19639,#19640);
#15861=AXIS2_PLACEMENT_3D('',#25299,#19642,#19643);
#15862=AXIS2_PLACEMENT_3D('',#25301,#19645,#19646);
#15863=AXIS2_PLACEMENT_3D('',#25303,#19648,#19649);
#15864=AXIS2_PLACEMENT_3D('',#25305,#19651,#19652);
#15865=AXIS2_PLACEMENT_3D('',#25307,#19654,#19655);
#15866=AXIS2_PLACEMENT_3D('',#25309,#19657,#19658);
#15867=AXIS2_PLACEMENT_3D('',#25311,#19660,#19661);
#15868=AXIS2_PLACEMENT_3D('',#25313,#19663,#19664);
#15869=AXIS2_PLACEMENT_3D('',#25315,#19666,#19667);
#15870=AXIS2_PLACEMENT_3D('',#25317,#19669,#19670);
#19337=DIRECTION('axis',(0.,0.,1.));
#19338=DIRECTION('refdir',(1.,0.,0.));
#19339=DIRECTION('center_axis',(1.,0.,6.12323399573677E-17));
#19340=DIRECTION('ref_axis',(6.12323399573677E-17,0.,-1.));
#19341=DIRECTION('',(1.,0.,6.12323399573677E-17));
#19342=DIRECTION('center_axis',(1.,0.,6.12323399573677E-17));
#19343=DIRECTION('ref_axis',(6.12323399573677E-17,0.,-1.));
#19344=DIRECTION('',(1.,0.,6.12323399573677E-17));
#19345=DIRECTION('center_axis',(0.,-1.,0.));
#19346=DIRECTION('ref_axis',(1.,0.,0.));
#19347=DIRECTION('center_axis',(0.,-1.,0.));
#19348=DIRECTION('ref_axis',(1.,0.,0.));
#19349=DIRECTION('',(0.,1.,0.));
#19350=DIRECTION('',(0.,1.,0.));
#19351=DIRECTION('center_axis',(0.,1.,0.));
#19352=DIRECTION('ref_axis',(1.,0.,0.));
#19353=DIRECTION('center_axis',(0.,0.,1.));
#19354=DIRECTION('ref_axis',(1.,0.,0.));
#19355=DIRECTION('',(0.,0.,1.));
#19356=DIRECTION('center_axis',(0.,0.,1.));
#19357=DIRECTION('ref_axis',(1.,0.,0.));
#19358=DIRECTION('',(0.,0.,1.));
#19359=DIRECTION('center_axis',(0.,1.,0.));
#19360=DIRECTION('ref_axis',(1.,0.,0.));
#19361=DIRECTION('center_axis',(0.,1.,0.));
#19362=DIRECTION('ref_axis',(1.,0.,0.));
#19363=DIRECTION('',(0.,1.,0.));
#19364=DIRECTION('',(0.,1.,0.));
#19365=DIRECTION('center_axis',(0.,-1.,0.));
#19366=DIRECTION('ref_axis',(1.,0.,0.));
#19367=DIRECTION('center_axis',(0.,1.,0.));
#19368=DIRECTION('ref_axis',(1.,0.,0.));
#19369=DIRECTION('center_axis',(0.,1.,0.));
#19370=DIRECTION('ref_axis',(1.,0.,0.));
#19371=DIRECTION('center_axis',(0.,1.,0.));
#19372=DIRECTION('ref_axis',(1.,0.,0.));
#19373=DIRECTION('center_axis',(0.,1.,0.));
#19374=DIRECTION('ref_axis',(0.951056516295154,0.,0.309016994374948));
#19375=DIRECTION('center_axis',(0.,1.,0.));
#19376=DIRECTION('ref_axis',(1.,0.,0.));
#19377=DIRECTION('center_axis',(0.,1.,0.));
#19378=DIRECTION('ref_axis',(0.809016994374947,0.,0.587785252292473));
#19379=DIRECTION('center_axis',(0.,1.,0.));
#19380=DIRECTION('ref_axis',(1.,0.,0.));
#19381=DIRECTION('center_axis',(0.,1.,0.));
#19382=DIRECTION('ref_axis',(0.587785252292473,0.,0.809016994374948));
#19383=DIRECTION('center_axis',(0.,1.,0.));
#19384=DIRECTION('ref_axis',(1.,0.,0.));
#19385=DIRECTION('center_axis',(0.,1.,0.));
#19386=DIRECTION('ref_axis',(0.309016994374947,0.,0.951056516295154));
#19387=DIRECTION('center_axis',(0.,1.,0.));
#19388=DIRECTION('ref_axis',(1.,0.,0.));
#19389=DIRECTION('center_axis',(0.,1.,0.));
#19390=DIRECTION('ref_axis',(-1.83697019872103E-16,0.,1.));
#19391=DIRECTION('center_axis',(0.,1.,0.));
#19392=DIRECTION('ref_axis',(1.,0.,0.));
#19393=DIRECTION('center_axis',(0.,1.,0.));
#19394=DIRECTION('ref_axis',(-0.309016994374948,0.,0.951056516295154));
#19395=DIRECTION('center_axis',(0.,1.,0.));
#19396=DIRECTION('ref_axis',(1.,0.,0.));
#19397=DIRECTION('center_axis',(0.,1.,0.));
#19398=DIRECTION('ref_axis',(-0.587785252292473,0.,0.809016994374947));
#19399=DIRECTION('center_axis',(0.,1.,0.));
#19400=DIRECTION('ref_axis',(1.,0.,0.));
#19401=DIRECTION('center_axis',(0.,1.,0.));
#19402=DIRECTION('ref_axis',(-0.809016994374947,0.,0.587785252292473));
#19403=DIRECTION('center_axis',(0.,1.,0.));
#19404=DIRECTION('ref_axis',(1.,0.,0.));
#19405=DIRECTION('center_axis',(0.,1.,0.));
#19406=DIRECTION('ref_axis',(-0.951056516295154,0.,0.309016994374947));
#19407=DIRECTION('center_axis',(0.,1.,0.));
#19408=DIRECTION('ref_axis',(1.,0.,0.));
#19409=DIRECTION('center_axis',(0.,1.,0.));
#19410=DIRECTION('ref_axis',(-1.,0.,-1.22464679914735E-16));
#19411=DIRECTION('center_axis',(0.,1.,0.));
#19412=DIRECTION('ref_axis',(1.,0.,0.));
#19413=DIRECTION('center_axis',(0.,1.,0.));
#19414=DIRECTION('ref_axis',(-0.951056516295154,0.,-0.309016994374948));
#19415=DIRECTION('center_axis',(0.,1.,0.));
#19416=DIRECTION('ref_axis',(1.,0.,0.));
#19417=DIRECTION('center_axis',(0.,1.,0.));
#19418=DIRECTION('ref_axis',(-0.809016994374947,0.,-0.587785252292473));
#19419=DIRECTION('center_axis',(0.,1.,0.));
#19420=DIRECTION('ref_axis',(1.,0.,0.));
#19421=DIRECTION('center_axis',(0.,1.,0.));
#19422=DIRECTION('ref_axis',(-0.587785252292473,0.,-0.809016994374948));
#19423=DIRECTION('center_axis',(0.,1.,0.));
#19424=DIRECTION('ref_axis',(1.,0.,0.));
#19425=DIRECTION('center_axis',(0.,1.,0.));
#19426=DIRECTION('ref_axis',(-0.309016994374947,0.,-0.951056516295154));
#19427=DIRECTION('center_axis',(0.,1.,0.));
#19428=DIRECTION('ref_axis',(1.,0.,0.));
#19429=DIRECTION('center_axis',(0.,1.,0.));
#19430=DIRECTION('ref_axis',(6.12323399573677E-17,0.,-1.));
#19431=DIRECTION('center_axis',(0.,1.,0.));
#19432=DIRECTION('ref_axis',(1.,0.,0.));
#19433=DIRECTION('center_axis',(0.,1.,0.));
#19434=DIRECTION('ref_axis',(0.309016994374947,0.,-0.951056516295154));
#19435=DIRECTION('center_axis',(0.,1.,0.));
#19436=DIRECTION('ref_axis',(1.,0.,0.));
#19437=DIRECTION('center_axis',(0.,1.,0.));
#19438=DIRECTION('ref_axis',(0.587785252292473,0.,-0.809016994374947));
#19439=DIRECTION('center_axis',(0.,1.,0.));
#19440=DIRECTION('ref_axis',(1.,0.,0.));
#19441=DIRECTION('center_axis',(0.,1.,0.));
#19442=DIRECTION('ref_axis',(0.809016994374947,0.,-0.587785252292473));
#19443=DIRECTION('center_axis',(0.,1.,0.));
#19444=DIRECTION('ref_axis',(1.,0.,0.));
#19445=DIRECTION('center_axis',(0.,1.,0.));
#19446=DIRECTION('ref_axis',(0.951056516295154,0.,-0.309016994374947));
#19447=DIRECTION('center_axis',(0.,1.,0.));
#19448=DIRECTION('ref_axis',(1.,0.,0.));
#19449=DIRECTION('center_axis',(0.,1.,0.));
#19450=DIRECTION('ref_axis',(1.,0.,0.));
#19451=DIRECTION('center_axis',(0.,1.,0.));
#19452=DIRECTION('ref_axis',(1.,0.,0.));
#19453=DIRECTION('center_axis',(0.,-1.,0.));
#19454=DIRECTION('ref_axis',(1.,0.,0.));
#19455=DIRECTION('center_axis',(0.,-1.,0.));
#19456=DIRECTION('ref_axis',(1.,0.,0.));
#19457=DIRECTION('',(0.,1.,0.));
#19458=DIRECTION('center_axis',(0.,1.,0.));
#19459=DIRECTION('ref_axis',(1.,0.,0.));
#19460=DIRECTION('center_axis',(0.,1.,0.));
#19461=DIRECTION('ref_axis',(1.,0.,0.));
#19462=DIRECTION('center_axis',(0.,1.,0.));
#19463=DIRECTION('ref_axis',(1.,0.,0.));
#19464=DIRECTION('center_axis',(0.,-1.,0.));
#19465=DIRECTION('ref_axis',(0.951056516295154,0.,0.309016994374948));
#19466=DIRECTION('center_axis',(0.,1.,0.));
#19467=DIRECTION('ref_axis',(1.,0.,0.));
#19468=DIRECTION('center_axis',(0.,-1.,0.));
#19469=DIRECTION('ref_axis',(1.,0.,0.));
#19470=DIRECTION('center_axis',(0.,1.,0.));
#19471=DIRECTION('ref_axis',(1.,0.,0.));
#19472=DIRECTION('center_axis',(0.,-1.,0.));
#19473=DIRECTION('ref_axis',(0.951056516295154,0.,-0.309016994374947));
#19474=DIRECTION('center_axis',(0.,1.,0.));
#19475=DIRECTION('ref_axis',(1.,0.,0.));
#19476=DIRECTION('center_axis',(0.,-1.,0.));
#19477=DIRECTION('ref_axis',(0.809016994374947,0.,-0.587785252292473));
#19478=DIRECTION('center_axis',(0.,1.,0.));
#19479=DIRECTION('ref_axis',(1.,0.,0.));
#19480=DIRECTION('center_axis',(0.,-1.,0.));
#19481=DIRECTION('ref_axis',(0.587785252292473,0.,-0.809016994374947));
#19482=DIRECTION('center_axis',(0.,1.,0.));
#19483=DIRECTION('ref_axis',(1.,0.,0.));
#19484=DIRECTION('center_axis',(0.,-1.,0.));
#19485=DIRECTION('ref_axis',(0.309016994374947,0.,-0.951056516295154));
#19486=DIRECTION('center_axis',(0.,1.,0.));
#19487=DIRECTION('ref_axis',(1.,0.,0.));
#19488=DIRECTION('center_axis',(0.,-1.,0.));
#19489=DIRECTION('ref_axis',(6.12323399573677E-17,0.,-1.));
#19490=DIRECTION('center_axis',(0.,1.,0.));
#19491=DIRECTION('ref_axis',(1.,0.,0.));
#19492=DIRECTION('center_axis',(0.,-1.,0.));
#19493=DIRECTION('ref_axis',(-0.309016994374947,0.,-0.951056516295154));
#19494=DIRECTION('center_axis',(0.,1.,0.));
#19495=DIRECTION('ref_axis',(1.,0.,0.));
#19496=DIRECTION('center_axis',(0.,-1.,0.));
#19497=DIRECTION('ref_axis',(-0.587785252292473,0.,-0.809016994374948));
#19498=DIRECTION('center_axis',(0.,1.,0.));
#19499=DIRECTION('ref_axis',(1.,0.,0.));
#19500=DIRECTION('center_axis',(0.,-1.,0.));
#19501=DIRECTION('ref_axis',(-0.809016994374947,0.,-0.587785252292473));
#19502=DIRECTION('center_axis',(0.,1.,0.));
#19503=DIRECTION('ref_axis',(1.,0.,0.));
#19504=DIRECTION('center_axis',(0.,-1.,0.));
#19505=DIRECTION('ref_axis',(-0.951056516295154,0.,-0.309016994374948));
#19506=DIRECTION('center_axis',(0.,1.,0.));
#19507=DIRECTION('ref_axis',(1.,0.,0.));
#19508=DIRECTION('center_axis',(0.,-1.,0.));
#19509=DIRECTION('ref_axis',(-1.,0.,-1.22464679914735E-16));
#19510=DIRECTION('center_axis',(0.,1.,0.));
#19511=DIRECTION('ref_axis',(1.,0.,0.));
#19512=DIRECTION('center_axis',(0.,-1.,0.));
#19513=DIRECTION('ref_axis',(-0.951056516295154,0.,0.309016994374947));
#19514=DIRECTION('center_axis',(0.,1.,0.));
#19515=DIRECTION('ref_axis',(1.,0.,0.));
#19516=DIRECTION('center_axis',(0.,-1.,0.));
#19517=DIRECTION('ref_axis',(-0.809016994374947,0.,0.587785252292473));
#19518=DIRECTION('center_axis',(0.,1.,0.));
#19519=DIRECTION('ref_axis',(1.,0.,0.));
#19520=DIRECTION('center_axis',(0.,-1.,0.));
#19521=DIRECTION('ref_axis',(-0.587785252292473,0.,0.809016994374947));
#19522=DIRECTION('center_axis',(0.,1.,0.));
#19523=DIRECTION('ref_axis',(1.,0.,0.));
#19524=DIRECTION('center_axis',(0.,-1.,0.));
#19525=DIRECTION('ref_axis',(-0.309016994374948,0.,0.951056516295154));
#19526=DIRECTION('center_axis',(0.,1.,0.));
#19527=DIRECTION('ref_axis',(1.,0.,0.));
#19528=DIRECTION('center_axis',(0.,-1.,0.));
#19529=DIRECTION('ref_axis',(-1.83697019872103E-16,0.,1.));
#19530=DIRECTION('center_axis',(0.,1.,0.));
#19531=DIRECTION('ref_axis',(1.,0.,0.));
#19532=DIRECTION('center_axis',(0.,-1.,0.));
#19533=DIRECTION('ref_axis',(0.309016994374947,0.,0.951056516295154));
#19534=DIRECTION('center_axis',(0.,1.,0.));
#19535=DIRECTION('ref_axis',(1.,0.,0.));
#19536=DIRECTION('center_axis',(0.,-1.,0.));
#19537=DIRECTION('ref_axis',(0.587785252292473,0.,0.809016994374948));
#19538=DIRECTION('center_axis',(0.,1.,0.));
#19539=DIRECTION('ref_axis',(1.,0.,0.));
#19540=DIRECTION('center_axis',(0.,-1.,0.));
#19541=DIRECTION('ref_axis',(0.809016994374947,0.,0.587785252292473));
#19542=DIRECTION('center_axis',(0.,1.,0.));
#19543=DIRECTION('ref_axis',(1.,0.,0.));
#19544=DIRECTION('center_axis',(0.,1.,0.));
#19545=DIRECTION('ref_axis',(1.,0.,0.));
#19546=DIRECTION('center_axis',(0.,1.,0.));
#19547=DIRECTION('ref_axis',(1.,0.,0.));
#19548=DIRECTION('',(0.,-1.,0.));
#19549=DIRECTION('center_axis',(0.,1.,0.));
#19550=DIRECTION('ref_axis',(1.,0.,0.));
#19551=DIRECTION('center_axis',(0.,1.,0.));
#19552=DIRECTION('ref_axis',(-0.951056516295153,0.,-0.309016994374948));
#19553=DIRECTION('',(0.,-1.,0.));
#19554=DIRECTION('',(0.,1.,0.));
#19555=DIRECTION('center_axis',(0.,1.,0.));
#19556=DIRECTION('ref_axis',(1.,0.,0.));
#19557=DIRECTION('',(0.,-1.,0.));
#19558=DIRECTION('center_axis',(0.,1.,0.));
#19559=DIRECTION('ref_axis',(-0.809016994374947,0.,-0.587785252292473));
#19560=DIRECTION('',(0.,1.,0.));
#19561=DIRECTION('center_axis',(0.,1.,0.));
#19562=DIRECTION('ref_axis',(1.,0.,0.));
#19563=DIRECTION('',(0.,-1.,0.));
#19564=DIRECTION('center_axis',(0.,1.,0.));
#19565=DIRECTION('ref_axis',(-0.587785252292473,0.,-0.809016994374947));
#19566=DIRECTION('',(0.,1.,0.));
#19567=DIRECTION('center_axis',(0.,1.,0.));
#19568=DIRECTION('ref_axis',(1.,0.,0.));
#19569=DIRECTION('',(0.,-1.,0.));
#19570=DIRECTION('center_axis',(0.,1.,0.));
#19571=DIRECTION('ref_axis',(-0.309016994374947,0.,-0.951056516295154));
#19572=DIRECTION('',(0.,1.,0.));
#19573=DIRECTION('center_axis',(0.,1.,0.));
#19574=DIRECTION('ref_axis',(1.,0.,0.));
#19575=DIRECTION('',(0.,-1.,0.));
#19576=DIRECTION('center_axis',(0.,1.,0.));
#19577=DIRECTION('ref_axis',(-1.37927510063224E-16,0.,-1.));
#19578=DIRECTION('',(0.,1.,0.));
#19579=DIRECTION('center_axis',(0.,1.,0.));
#19580=DIRECTION('ref_axis',(1.,0.,0.));
#19581=DIRECTION('',(0.,-1.,0.));
#19582=DIRECTION('center_axis',(0.,1.,0.));
#19583=DIRECTION('ref_axis',(0.309016994374948,0.,-0.951056516295154));
#19584=DIRECTION('',(0.,1.,0.));
#19585=DIRECTION('center_axis',(0.,1.,0.));
#19586=DIRECTION('ref_axis',(1.,0.,0.));
#19587=DIRECTION('',(0.,-1.,0.));
#19588=DIRECTION('center_axis',(0.,1.,0.));
#19589=DIRECTION('ref_axis',(0.587785252292473,0.,-0.809016994374948));
#19590=DIRECTION('',(0.,1.,0.));
#19591=DIRECTION('center_axis',(0.,1.,0.));
#19592=DIRECTION('ref_axis',(1.,0.,0.));
#19593=DIRECTION('',(0.,-1.,0.));
#19594=DIRECTION('center_axis',(0.,1.,0.));
#19595=DIRECTION('ref_axis',(0.809016994374948,0.,-0.587785252292473));
#19596=DIRECTION('',(0.,1.,0.));
#19597=DIRECTION('center_axis',(0.,1.,0.));
#19598=DIRECTION('ref_axis',(1.,0.,0.));
#19599=DIRECTION('',(0.,-1.,0.));
#19600=DIRECTION('center_axis',(0.,1.,0.));
#19601=DIRECTION('ref_axis',(0.951056516295154,0.,-0.309016994374947));
#19602=DIRECTION('',(0.,1.,0.));
#19603=DIRECTION('center_axis',(0.,1.,0.));
#19604=DIRECTION('ref_axis',(1.,0.,0.));
#19605=DIRECTION('',(0.,-1.,0.));
#19606=DIRECTION('center_axis',(0.,1.,0.));
#19607=DIRECTION('ref_axis',(1.,0.,-1.99159850020592E-16));
#19608=DIRECTION('',(0.,1.,0.));
#19609=DIRECTION('center_axis',(0.,1.,0.));
#19610=DIRECTION('ref_axis',(1.,0.,0.));
#19611=DIRECTION('',(0.,-1.,0.));
#19612=DIRECTION('center_axis',(0.,1.,0.));
#19613=DIRECTION('ref_axis',(0.951056516295154,0.,0.309016994374948));
#19614=DIRECTION('',(0.,1.,0.));
#19615=DIRECTION('center_axis',(0.,1.,0.));
#19616=DIRECTION('ref_axis',(1.,0.,0.));
#19617=DIRECTION('',(0.,-1.,0.));
#19618=DIRECTION('center_axis',(0.,1.,0.));
#19619=DIRECTION('ref_axis',(0.809016994374948,0.,0.587785252292473));
#19620=DIRECTION('',(0.,1.,0.));
#19621=DIRECTION('center_axis',(0.,1.,0.));
#19622=DIRECTION('ref_axis',(1.,0.,0.));
#19623=DIRECTION('',(0.,-1.,0.));
#19624=DIRECTION('center_axis',(0.,1.,0.));
#19625=DIRECTION('ref_axis',(0.587785252292473,0.,0.809016994374948));
#19626=DIRECTION('',(0.,1.,0.));
#19627=DIRECTION('center_axis',(0.,1.,0.));
#19628=DIRECTION('ref_axis',(1.,0.,0.));
#19629=DIRECTION('',(0.,-1.,0.));
#19630=DIRECTION('center_axis',(0.,1.,0.));
#19631=DIRECTION('ref_axis',(0.309016994374947,0.,0.951056516295154));
#19632=DIRECTION('',(0.,1.,0.));
#19633=DIRECTION('center_axis',(0.,1.,0.));
#19634=DIRECTION('ref_axis',(1.,0.,0.));
#19635=DIRECTION('',(0.,-1.,0.));
#19636=DIRECTION('center_axis',(0.,1.,0.));
#19637=DIRECTION('ref_axis',(2.6039218997796E-16,0.,1.));
#19638=DIRECTION('',(0.,1.,0.));
#19639=DIRECTION('center_axis',(0.,1.,0.));
#19640=DIRECTION('ref_axis',(1.,0.,0.));
#19641=DIRECTION('',(0.,-1.,0.));
#19642=DIRECTION('center_axis',(0.,1.,0.));
#19643=DIRECTION('ref_axis',(-0.309016994374948,0.,0.951056516295153));
#19644=DIRECTION('',(0.,1.,0.));
#19645=DIRECTION('center_axis',(0.,1.,0.));
#19646=DIRECTION('ref_axis',(1.,0.,0.));
#19647=DIRECTION('',(0.,-1.,0.));
#19648=DIRECTION('center_axis',(0.,1.,0.));
#19649=DIRECTION('ref_axis',(-0.587785252292474,0.,0.809016994374947));
#19650=DIRECTION('',(0.,1.,0.));
#19651=DIRECTION('center_axis',(0.,1.,0.));
#19652=DIRECTION('ref_axis',(1.,0.,0.));
#19653=DIRECTION('',(0.,-1.,0.));
#19654=DIRECTION('center_axis',(0.,1.,0.));
#19655=DIRECTION('ref_axis',(-0.809016994374948,0.,0.587785252292473));
#19656=DIRECTION('',(0.,1.,0.));
#19657=DIRECTION('center_axis',(0.,1.,0.));
#19658=DIRECTION('ref_axis',(1.,0.,0.));
#19659=DIRECTION('',(0.,-1.,0.));
#19660=DIRECTION('center_axis',(0.,1.,0.));
#19661=DIRECTION('ref_axis',(-0.951056516295154,0.,0.309016994374948));
#19662=DIRECTION('',(0.,1.,0.));
#19663=DIRECTION('center_axis',(0.,1.,0.));
#19664=DIRECTION('ref_axis',(1.,0.,0.));
#19665=DIRECTION('',(0.,1.,0.));
#19666=DIRECTION('center_axis',(0.,1.,0.));
#19667=DIRECTION('ref_axis',(-1.,0.,-1.22464679914735E-16));
#19668=DIRECTION('',(0.,-1.,0.));
#19669=DIRECTION('center_axis',(0.,1.,0.));
#19670=DIRECTION('ref_axis',(1.,0.,0.));
#24716=CARTESIAN_POINT('',(0.,0.,0.));
#24717=CARTESIAN_POINT('Origin',(0.,-0.45,0.));
#24718=CARTESIAN_POINT('',(-0.65,-0.325,-3.9801020972289E-17));
#24719=CARTESIAN_POINT('',(-0.637867541108654,-0.45,0.125));
#24720=CARTESIAN_POINT('Ctrl Pts',(-0.65,-0.325,-6.93889390390723E-17));
#24721=CARTESIAN_POINT('Ctrl Pts',(-0.65,-0.325,0.0157371373481997));
#24722=CARTESIAN_POINT('Ctrl Pts',(-0.649370620646074,-0.328153081062251,
0.0324967135411163));
#24723=CARTESIAN_POINT('Ctrl Pts',(-0.647096224417991,-0.340922081922822,
0.0632828231545122));
#24724=CARTESIAN_POINT('Ctrl Pts',(-0.645482573914132,-0.350535859112198,
0.0773125544088347));
#24725=CARTESIAN_POINT('Ctrl Pts',(-0.642442040715078,-0.372687974598127,
0.0994646698947638));
#24726=CARTESIAN_POINT('Ctrl Pts',(-0.640815160902589,-0.386717480603274,
0.109078032552995));
#24727=CARTESIAN_POINT('Ctrl Pts',(-0.63851034608138,-0.417502809542363,
0.121846732641678));
#24728=CARTESIAN_POINT('Ctrl Pts',(-0.637867541108654,-0.434262111007648,
0.125));
#24729=CARTESIAN_POINT('Ctrl Pts',(-0.637867541108654,-0.45,0.125));
#24730=CARTESIAN_POINT('',(-0.65,-0.575,-3.9801020972289E-17));
#24731=CARTESIAN_POINT('Ctrl Pts',(-0.65,-0.575,-3.46944695195361E-18));
#24732=CARTESIAN_POINT('Ctrl Pts',(-0.65,-0.575,-0.0157371373481998));
#24733=CARTESIAN_POINT('Ctrl Pts',(-0.649370620646074,-0.571846918937749,
-0.0324967135411164));
#24734=CARTESIAN_POINT('Ctrl Pts',(-0.647096224417991,-0.559077918077178,
-0.0632828231545123));
#24735=CARTESIAN_POINT('Ctrl Pts',(-0.645482573914132,-0.549464140887802,
-0.0773125544088349));
#24736=CARTESIAN_POINT('Ctrl Pts',(-0.642442040715078,-0.527312025401873,
-0.099464669894764));
#24737=CARTESIAN_POINT('Ctrl Pts',(-0.640815160902589,-0.513282519396725,
-0.109078032552995));
#24738=CARTESIAN_POINT('Ctrl Pts',(-0.63851034608138,-0.482497190457637,
-0.121846732641678));
#24739=CARTESIAN_POINT('Ctrl Pts',(-0.637867541108654,-0.465737888992352,
-0.125));
#24740=CARTESIAN_POINT('Ctrl Pts',(-0.637867541108654,-0.434262111007648,
-0.125));
#24741=CARTESIAN_POINT('Ctrl Pts',(-0.63851034608138,-0.417502809542363,
-0.121846732641678));
#24742=CARTESIAN_POINT('Ctrl Pts',(-0.640815160902589,-0.386717480603275,
-0.109078032552995));
#24743=CARTESIAN_POINT('Ctrl Pts',(-0.642442040715078,-0.372687974598127,
-0.099464669894764));
#24744=CARTESIAN_POINT('Ctrl Pts',(-0.645482573914132,-0.350535859112198,
-0.077312554408835));
#24745=CARTESIAN_POINT('Ctrl Pts',(-0.647096224417991,-0.340922081922822,
-0.0632828231545124));
#24746=CARTESIAN_POINT('Ctrl Pts',(-0.649370620646074,-0.328153081062251,
-0.0324967135411165));
#24747=CARTESIAN_POINT('Ctrl Pts',(-0.65,-0.325,-0.0157371373481999));
#24748=CARTESIAN_POINT('Ctrl Pts',(-0.65,-0.325,-8.32667268468867E-17));
#24749=CARTESIAN_POINT('Ctrl Pts',(-0.637867541108654,-0.45,0.125));
#24750=CARTESIAN_POINT('Ctrl Pts',(-0.637867541108654,-0.465737888992352,
0.125));
#24751=CARTESIAN_POINT('Ctrl Pts',(-0.63851034608138,-0.482497190457637,
0.121846732641678));
#24752=CARTESIAN_POINT('Ctrl Pts',(-0.640815160902589,-0.513282519396725,
0.109078032552995));
#24753=CARTESIAN_POINT('Ctrl Pts',(-0.642442040715078,-0.527312025401873,
0.0994646698947639));
#24754=CARTESIAN_POINT('Ctrl Pts',(-0.645482573914132,-0.549464140887802,
0.0773125544088349));
#24755=CARTESIAN_POINT('Ctrl Pts',(-0.647096224417991,-0.559077918077178,
0.0632828231545123));
#24756=CARTESIAN_POINT('Ctrl Pts',(-0.649370620646074,-0.571846918937749,
0.0324967135411164));
#24757=CARTESIAN_POINT('Ctrl Pts',(-0.65,-0.575,0.0157371373481998));
#24758=CARTESIAN_POINT('Ctrl Pts',(-0.65,-0.575,-2.08166817117217E-17));
#24759=CARTESIAN_POINT('',(-0.379967103839267,-0.45,0.125));
#24760=CARTESIAN_POINT('',(-7.65404249467096E-18,-0.45,0.125));
#24761=CARTESIAN_POINT('',(-0.4,-0.575,5.41097774720219E-18));
#24762=CARTESIAN_POINT('Ctrl Pts',(-0.4,-0.575,-3.81639164714898E-17));
#24763=CARTESIAN_POINT('Ctrl Pts',(-0.4,-0.575,0.0158075115832675));
#24764=CARTESIAN_POINT('Ctrl Pts',(-0.398970551469948,-0.571819306519379,
0.0325978607437828));
#24765=CARTESIAN_POINT('Ctrl Pts',(-0.395252954914593,-0.559029081159106,
0.0633657881355917));
#24766=CARTESIAN_POINT('Ctrl Pts',(-0.392612801026882,-0.549425200318011,
0.0773514949786256));
#24767=CARTESIAN_POINT('Ctrl Pts',(-0.38761064154154,-0.527347592689753,
0.0994291026068839));
#24768=CARTESIAN_POINT('Ctrl Pts',(-0.384911758361269,-0.51336346023721,
0.109029967924066));
#24769=CARTESIAN_POINT('Ctrl Pts',(-0.381057715344782,-0.48260129709332,
0.121817958968287));
#24770=CARTESIAN_POINT('Ctrl Pts',(-0.379967103839267,-0.465813100629203,
0.125));
#24771=CARTESIAN_POINT('Ctrl Pts',(-0.379967103839267,-0.45,0.125));
#24772=CARTESIAN_POINT('',(-0.379967103839267,-0.45,-0.125));
#24773=CARTESIAN_POINT('Ctrl Pts',(-0.379967103839267,-0.45,-0.125));
#24774=CARTESIAN_POINT('Ctrl Pts',(-0.379967103839267,-0.465813100629203,
-0.125));
#24775=CARTESIAN_POINT('Ctrl Pts',(-0.381057715344782,-0.48260129709332,
-0.121817958968287));
#24776=CARTESIAN_POINT('Ctrl Pts',(-0.384911758361269,-0.51336346023721,
-0.109029967924066));
#24777=CARTESIAN_POINT('Ctrl Pts',(-0.38761064154154,-0.527347592689753,
-0.099429102606884));
#24778=CARTESIAN_POINT('Ctrl Pts',(-0.392612801026882,-0.549425200318011,
-0.0773514949786257));
#24779=CARTESIAN_POINT('Ctrl Pts',(-0.395252954914593,-0.559029081159106,
-0.0633657881355918));
#24780=CARTESIAN_POINT('Ctrl Pts',(-0.398970551469948,-0.571819306519379,
-0.0325978607437828));
#24781=CARTESIAN_POINT('Ctrl Pts',(-0.4,-0.575,-0.0158075115832676));
#24782=CARTESIAN_POINT('Ctrl Pts',(-0.4,-0.575,-4.16333634234434E-17));
#24783=CARTESIAN_POINT('',(-0.4,-0.325,2.96971064108775E-17));
#24784=CARTESIAN_POINT('Ctrl Pts',(-0.4,-0.325,1.04083408558608E-17));
#24785=CARTESIAN_POINT('Ctrl Pts',(-0.4,-0.325,-0.0158075115832676));
#24786=CARTESIAN_POINT('Ctrl Pts',(-0.398970551469948,-0.328180693480621,
-0.0325978607437828));
#24787=CARTESIAN_POINT('Ctrl Pts',(-0.395252954914593,-0.340970918840894,
-0.0633657881355918));
#24788=CARTESIAN_POINT('Ctrl Pts',(-0.392612801026882,-0.350574799681989,
-0.0773514949786256));
#24789=CARTESIAN_POINT('Ctrl Pts',(-0.38761064154154,-0.372652407310247,
-0.0994291026068839));
#24790=CARTESIAN_POINT('Ctrl Pts',(-0.384911758361269,-0.38663653976279,
-0.109029967924066));
#24791=CARTESIAN_POINT('Ctrl Pts',(-0.381057715344782,-0.41739870290668,
-0.121817958968287));
#24792=CARTESIAN_POINT('Ctrl Pts',(-0.379967103839267,-0.434186899370797,
-0.125));
#24793=CARTESIAN_POINT('Ctrl Pts',(-0.379967103839267,-0.45,-0.125));
#24794=CARTESIAN_POINT('Ctrl Pts',(-0.379967103839267,-0.45,0.125));
#24795=CARTESIAN_POINT('Ctrl Pts',(-0.379967103839267,-0.434186899370797,
0.125));
#24796=CARTESIAN_POINT('Ctrl Pts',(-0.381057715344782,-0.41739870290668,
0.121817958968287));
#24797=CARTESIAN_POINT('Ctrl Pts',(-0.384911758361269,-0.38663653976279,
0.109029967924066));
#24798=CARTESIAN_POINT('Ctrl Pts',(-0.38761064154154,-0.372652407310247,
0.0994291026068839));
#24799=CARTESIAN_POINT('Ctrl Pts',(-0.392612801026882,-0.350574799681989,
0.0773514949786257));
#24800=CARTESIAN_POINT('Ctrl Pts',(-0.395252954914593,-0.340970918840894,
0.0633657881355918));
#24801=CARTESIAN_POINT('Ctrl Pts',(-0.398970551469948,-0.328180693480621,
0.0325978607437829));
#24802=CARTESIAN_POINT('Ctrl Pts',(-0.4,-0.325,0.0158075115832676));
#24803=CARTESIAN_POINT('Ctrl Pts',(-0.4,-0.325,1.38777878078145E-17));
#24804=CARTESIAN_POINT('Origin',(0.,-0.45,0.));
#24805=CARTESIAN_POINT('',(0.379967103839267,-0.45,-0.125));
#24806=CARTESIAN_POINT('',(0.379967103839267,-0.45,0.125));
#24807=CARTESIAN_POINT('Ctrl Pts',(0.379967103839267,-0.45,-0.125));
#24808=CARTESIAN_POINT('Ctrl Pts',(0.379967103839267,-0.434186899370797,
-0.125));
#24809=CARTESIAN_POINT('Ctrl Pts',(0.381057715344782,-0.41739870290668,
-0.121817958968287));
#24810=CARTESIAN_POINT('Ctrl Pts',(0.384911758361269,-0.38663653976279,
-0.109029967924066));
#24811=CARTESIAN_POINT('Ctrl Pts',(0.38761064154154,-0.372652407310247,
-0.0994291026068839));
#24812=CARTESIAN_POINT('Ctrl Pts',(0.392612801026882,-0.350574799681989,
-0.0773514949786256));
#24813=CARTESIAN_POINT('Ctrl Pts',(0.395252954914593,-0.340970918840894,
-0.0633657881355917));
#24814=CARTESIAN_POINT('Ctrl Pts',(0.398970551469948,-0.328180693480621,
-0.0325978607437828));
#24815=CARTESIAN_POINT('Ctrl Pts',(0.4,-0.325,-0.0158075115832675));
#24816=CARTESIAN_POINT('Ctrl Pts',(0.4,-0.325,0.0158075115832676));
#24817=CARTESIAN_POINT('Ctrl Pts',(0.398970551469948,-0.328180693480621,
0.0325978607437829));
#24818=CARTESIAN_POINT('Ctrl Pts',(0.395252954914593,-0.340970918840894,
0.0633657881355918));
#24819=CARTESIAN_POINT('Ctrl Pts',(0.392612801026882,-0.350574799681989,
0.0773514949786257));
#24820=CARTESIAN_POINT('Ctrl Pts',(0.38761064154154,-0.372652407310247,
0.099429102606884));
#24821=CARTESIAN_POINT('Ctrl Pts',(0.384911758361269,-0.38663653976279,
0.109029967924066));
#24822=CARTESIAN_POINT('Ctrl Pts',(0.381057715344782,-0.41739870290668,
0.121817958968287));
#24823=CARTESIAN_POINT('Ctrl Pts',(0.379967103839267,-0.434186899370797,
0.125));
#24824=CARTESIAN_POINT('Ctrl Pts',(0.379967103839267,-0.45,0.125));
#24825=CARTESIAN_POINT('Ctrl Pts',(0.379967103839267,-0.45,0.125));
#24826=CARTESIAN_POINT('Ctrl Pts',(0.379967103839267,-0.465813100629203,
0.125));
#24827=CARTESIAN_POINT('Ctrl Pts',(0.381057715344782,-0.48260129709332,
0.121817958968287));
#24828=CARTESIAN_POINT('Ctrl Pts',(0.384911758361269,-0.51336346023721,
0.109029967924066));
#24829=CARTESIAN_POINT('Ctrl Pts',(0.38761064154154,-0.527347592689753,
0.0994291026068839));
#24830=CARTESIAN_POINT('Ctrl Pts',(0.392612801026882,-0.549425200318011,
0.0773514949786257));
#24831=CARTESIAN_POINT('Ctrl Pts',(0.395252954914593,-0.559029081159106,
0.0633657881355918));
#24832=CARTESIAN_POINT('Ctrl Pts',(0.398970551469948,-0.571819306519379,
0.0325978607437829));
#24833=CARTESIAN_POINT('Ctrl Pts',(0.4,-0.575,0.0158075115832676));
#24834=CARTESIAN_POINT('Ctrl Pts',(0.4,-0.575,-0.0158075115832676));
#24835=CARTESIAN_POINT('Ctrl Pts',(0.398970551469948,-0.57181930651938,
-0.0325978607437828));
#24836=CARTESIAN_POINT('Ctrl Pts',(0.395252954914593,-0.559029081159106,
-0.0633657881355918));
#24837=CARTESIAN_POINT('Ctrl Pts',(0.392612801026882,-0.549425200318011,
-0.0773514949786257));
#24838=CARTESIAN_POINT('Ctrl Pts',(0.38761064154154,-0.527347592689753,
-0.0994291026068839));
#24839=CARTESIAN_POINT('Ctrl Pts',(0.384911758361269,-0.51336346023721,
-0.109029967924066));
#24840=CARTESIAN_POINT('Ctrl Pts',(0.381057715344782,-0.48260129709332,
-0.121817958968287));
#24841=CARTESIAN_POINT('Ctrl Pts',(0.379967103839267,-0.465813100629203,
-0.125));
#24842=CARTESIAN_POINT('Ctrl Pts',(0.379967103839267,-0.45,-0.125));
#24843=CARTESIAN_POINT('',(0.637867541108654,-0.45,0.125));
#24844=CARTESIAN_POINT('',(-7.65404249467096E-18,-0.45,0.125));
#24845=CARTESIAN_POINT('',(0.65,-0.575,3.9801020972289E-17));
#24846=CARTESIAN_POINT('Ctrl Pts',(0.65,-0.575,5.55111512312578E-17));
#24847=CARTESIAN_POINT('Ctrl Pts',(0.65,-0.575,0.0157371373481999));
#24848=CARTESIAN_POINT('Ctrl Pts',(0.649370620646074,-0.571846918937749,
0.0324967135411165));
#24849=CARTESIAN_POINT('Ctrl Pts',(0.647096224417991,-0.559077918077178,
0.0632828231545124));
#24850=CARTESIAN_POINT('Ctrl Pts',(0.645482573914132,-0.549464140887802,
0.077312554408835));
#24851=CARTESIAN_POINT('Ctrl Pts',(0.642442040715078,-0.527312025401873,
0.099464669894764));
#24852=CARTESIAN_POINT('Ctrl Pts',(0.640815160902589,-0.513282519396725,
0.109078032552995));
#24853=CARTESIAN_POINT('Ctrl Pts',(0.63851034608138,-0.482497190457637,
0.121846732641678));
#24854=CARTESIAN_POINT('Ctrl Pts',(0.637867541108654,-0.465737888992352,
0.125));
#24855=CARTESIAN_POINT('Ctrl Pts',(0.637867541108654,-0.45,0.125));
#24856=CARTESIAN_POINT('',(0.65,-0.325,3.9801020972289E-17));
#24857=CARTESIAN_POINT('Ctrl Pts',(0.65,-0.325,6.93889390390723E-18));
#24858=CARTESIAN_POINT('Ctrl Pts',(0.65,-0.325,-0.0157371373481998));
#24859=CARTESIAN_POINT('Ctrl Pts',(0.649370620646074,-0.328153081062251,
-0.0324967135411164));
#24860=CARTESIAN_POINT('Ctrl Pts',(0.647096224417991,-0.340922081922822,
-0.0632828231545123));
#24861=CARTESIAN_POINT('Ctrl Pts',(0.645482573914132,-0.350535859112198,
-0.0773125544088349));
#24862=CARTESIAN_POINT('Ctrl Pts',(0.642442040715078,-0.372687974598127,
-0.0994646698947639));
#24863=CARTESIAN_POINT('Ctrl Pts',(0.640815160902588,-0.386717480603275,
-0.109078032552995));
#24864=CARTESIAN_POINT('Ctrl Pts',(0.63851034608138,-0.417502809542363,
-0.121846732641678));
#24865=CARTESIAN_POINT('Ctrl Pts',(0.637867541108654,-0.434262111007648,
-0.125));
#24866=CARTESIAN_POINT('Ctrl Pts',(0.637867541108654,-0.465737888992352,
-0.125));
#24867=CARTESIAN_POINT('Ctrl Pts',(0.63851034608138,-0.482497190457637,
-0.121846732641678));
#24868=CARTESIAN_POINT('Ctrl Pts',(0.640815160902589,-0.513282519396725,
-0.109078032552995));
#24869=CARTESIAN_POINT('Ctrl Pts',(0.642442040715078,-0.527312025401873,
-0.0994646698947639));
#24870=CARTESIAN_POINT('Ctrl Pts',(0.645482573914132,-0.549464140887802,
-0.0773125544088348));
#24871=CARTESIAN_POINT('Ctrl Pts',(0.647096224417991,-0.559077918077178,
-0.0632828231545123));
#24872=CARTESIAN_POINT('Ctrl Pts',(0.649370620646074,-0.571846918937749,
-0.0324967135411164));
#24873=CARTESIAN_POINT('Ctrl Pts',(0.65,-0.575,-0.0157371373481998));
#24874=CARTESIAN_POINT('Ctrl Pts',(0.65,-0.575,6.24500451351651E-17));
#24875=CARTESIAN_POINT('Ctrl Pts',(0.637867541108654,-0.45,0.125));
#24876=CARTESIAN_POINT('Ctrl Pts',(0.637867541108654,-0.434262111007648,
0.125));
#24877=CARTESIAN_POINT('Ctrl Pts',(0.63851034608138,-0.417502809542363,
0.121846732641678));
#24878=CARTESIAN_POINT('Ctrl Pts',(0.640815160902589,-0.386717480603274,
0.109078032552995));
#24879=CARTESIAN_POINT('Ctrl Pts',(0.642442040715078,-0.372687974598127,
0.0994646698947639));
#24880=CARTESIAN_POINT('Ctrl Pts',(0.645482573914132,-0.350535859112198,
0.0773125544088348));
#24881=CARTESIAN_POINT('Ctrl Pts',(0.647096224417991,-0.340922081922822,
0.0632828231545123));
#24882=CARTESIAN_POINT('Ctrl Pts',(0.649370620646074,-0.328153081062251,
0.0324967135411164));
#24883=CARTESIAN_POINT('Ctrl Pts',(0.65,-0.325,0.0157371373481998));
#24884=CARTESIAN_POINT('Ctrl Pts',(0.65,-0.325,-6.93889390390723E-18));
#24885=CARTESIAN_POINT('Origin',(0.,-0.1,0.));
#24886=CARTESIAN_POINT('',(-0.65,-0.8,7.9602041944578E-17));
#24887=CARTESIAN_POINT('Origin',(0.,-0.8,0.));
#24888=CARTESIAN_POINT('',(-0.65,-0.1,-7.9602041944578E-17));
#24889=CARTESIAN_POINT('',(-0.65,-0.1,7.9602041944578E-17));
#24890=CARTESIAN_POINT('',(-0.65,-0.1,-7.9602041944578E-17));
#24891=CARTESIAN_POINT('Origin',(0.,-0.1,0.));
#24892=CARTESIAN_POINT('',(0.,-0.575,-0.65));
#24893=CARTESIAN_POINT('',(0.,-0.325,-0.65));
#24894=CARTESIAN_POINT('Ctrl Pts',(-1.73472347597681E-17,-0.575,-0.65));
#24895=CARTESIAN_POINT('Ctrl Pts',(0.0157371373481998,-0.575,-0.65));
#24896=CARTESIAN_POINT('Ctrl Pts',(0.0324967135411164,-0.571846918937749,
-0.649370620646074));
#24897=CARTESIAN_POINT('Ctrl Pts',(0.0632828231545123,-0.559077918077178,
-0.647096224417991));
#24898=CARTESIAN_POINT('Ctrl Pts',(0.0773125544088349,-0.549464140887802,
-0.645482573914132));
#24899=CARTESIAN_POINT('Ctrl Pts',(0.099464669894764,-0.527312025401873,
-0.642442040715078));
#24900=CARTESIAN_POINT('Ctrl Pts',(0.109078032552995,-0.513282519396725,
-0.640815160902589));
#24901=CARTESIAN_POINT('Ctrl Pts',(0.121846732641678,-0.482497190457636,
-0.63851034608138));
#24902=CARTESIAN_POINT('Ctrl Pts',(0.125,-0.465737888992352,-0.637867541108654));
#24903=CARTESIAN_POINT('Ctrl Pts',(0.125,-0.434262111007648,-0.637867541108654));
#24904=CARTESIAN_POINT('Ctrl Pts',(0.121846732641678,-0.417502809542364,
-0.63851034608138));
#24905=CARTESIAN_POINT('Ctrl Pts',(0.109078032552995,-0.386717480603275,
-0.640815160902589));
#24906=CARTESIAN_POINT('Ctrl Pts',(0.099464669894764,-0.372687974598127,
-0.642442040715078));
#24907=CARTESIAN_POINT('Ctrl Pts',(0.0773125544088349,-0.350535859112198,
-0.645482573914132));
#24908=CARTESIAN_POINT('Ctrl Pts',(0.0632828231545123,-0.340922081922822,
-0.647096224417991));
#24909=CARTESIAN_POINT('Ctrl Pts',(0.0324967135411164,-0.328153081062251,
-0.649370620646074));
#24910=CARTESIAN_POINT('Ctrl Pts',(0.0157371373481999,-0.325,-0.65));
#24911=CARTESIAN_POINT('Ctrl Pts',(4.5102810375397E-17,-0.325,-0.65));
#24912=CARTESIAN_POINT('',(-0.125,-0.45,-0.637867541108654));
#24913=CARTESIAN_POINT('Ctrl Pts',(4.85722573273506E-17,-0.325,-0.65));
#24914=CARTESIAN_POINT('Ctrl Pts',(-0.0157371373481997,-0.325,-0.65));
#24915=CARTESIAN_POINT('Ctrl Pts',(-0.0324967135411163,-0.328153081062251,
-0.649370620646074));
#24916=CARTESIAN_POINT('Ctrl Pts',(-0.0632828231545122,-0.340922081922822,
-0.647096224417991));
#24917=CARTESIAN_POINT('Ctrl Pts',(-0.0773125544088348,-0.350535859112198,
-0.645482573914132));
#24918=CARTESIAN_POINT('Ctrl Pts',(-0.0994646698947639,-0.372687974598127,
-0.642442040715078));
#24919=CARTESIAN_POINT('Ctrl Pts',(-0.109078032552995,-0.386717480603274,
-0.640815160902589));
#24920=CARTESIAN_POINT('Ctrl Pts',(-0.121846732641678,-0.417502809542363,
-0.63851034608138));
#24921=CARTESIAN_POINT('Ctrl Pts',(-0.125,-0.434262111007648,-0.637867541108654));
#24922=CARTESIAN_POINT('Ctrl Pts',(-0.125,-0.45,-0.637867541108654));
#24923=CARTESIAN_POINT('Ctrl Pts',(-0.125,-0.45,-0.637867541108654));
#24924=CARTESIAN_POINT('Ctrl Pts',(-0.125,-0.465737888992352,-0.637867541108654));
#24925=CARTESIAN_POINT('Ctrl Pts',(-0.121846732641678,-0.482497190457636,
-0.63851034608138));
#24926=CARTESIAN_POINT('Ctrl Pts',(-0.109078032552995,-0.513282519396725,
-0.640815160902589));
#24927=CARTESIAN_POINT('Ctrl Pts',(-0.099464669894764,-0.527312025401873,
-0.642442040715078));
#24928=CARTESIAN_POINT('Ctrl Pts',(-0.0773125544088349,-0.549464140887802,
-0.645482573914132));
#24929=CARTESIAN_POINT('Ctrl Pts',(-0.0632828231545124,-0.559077918077178,
-0.647096224417991));
#24930=CARTESIAN_POINT('Ctrl Pts',(-0.0324967135411165,-0.571846918937749,
-0.649370620646074));
#24931=CARTESIAN_POINT('Ctrl Pts',(-0.0157371373481998,-0.575,-0.65));
#24932=CARTESIAN_POINT('Ctrl Pts',(-1.73472347597681E-17,-0.575,-0.65));
#24933=CARTESIAN_POINT('',(0.,-0.325,0.65));
#24934=CARTESIAN_POINT('',(0.,-0.575,0.65));
#24935=CARTESIAN_POINT('Ctrl Pts',(2.77555756156289E-17,-0.325,0.65));
#24936=CARTESIAN_POINT('Ctrl Pts',(0.0157371373481998,-0.325,0.65));
#24937=CARTESIAN_POINT('Ctrl Pts',(0.0324967135411164,-0.328153081062251,
0.649370620646074));
#24938=CARTESIAN_POINT('Ctrl Pts',(0.0632828231545123,-0.340922081922822,
0.647096224417991));
#24939=CARTESIAN_POINT('Ctrl Pts',(0.0773125544088349,-0.350535859112198,
0.645482573914132));
#24940=CARTESIAN_POINT('Ctrl Pts',(0.099464669894764,-0.372687974598127,
0.642442040715078));
#24941=CARTESIAN_POINT('Ctrl Pts',(0.109078032552995,-0.386717480603275,
0.640815160902589));
#24942=CARTESIAN_POINT('Ctrl Pts',(0.121846732641678,-0.417502809542364,
0.63851034608138));
#24943=CARTESIAN_POINT('Ctrl Pts',(0.125,-0.434262111007648,0.637867541108654));
#24944=CARTESIAN_POINT('Ctrl Pts',(0.125,-0.465737888992352,0.637867541108654));
#24945=CARTESIAN_POINT('Ctrl Pts',(0.121846732641678,-0.482497190457636,
0.63851034608138));
#24946=CARTESIAN_POINT('Ctrl Pts',(0.109078032552995,-0.513282519396725,
0.640815160902589));
#24947=CARTESIAN_POINT('Ctrl Pts',(0.099464669894764,-0.527312025401873,
0.642442040715078));
#24948=CARTESIAN_POINT('Ctrl Pts',(0.077312554408835,-0.549464140887802,
0.645482573914132));
#24949=CARTESIAN_POINT('Ctrl Pts',(0.0632828231545124,-0.559077918077178,
0.647096224417991));
#24950=CARTESIAN_POINT('Ctrl Pts',(0.0324967135411165,-0.571846918937749,
0.649370620646074));
#24951=CARTESIAN_POINT('Ctrl Pts',(0.0157371373481998,-0.575,0.65));
#24952=CARTESIAN_POINT('Ctrl Pts',(-1.38777878078145E-17,-0.575,0.65));
#24953=CARTESIAN_POINT('',(-0.125,-0.45,0.637867541108654));
#24954=CARTESIAN_POINT('Ctrl Pts',(-1.04083408558608E-17,-0.575,0.65));
#24955=CARTESIAN_POINT('Ctrl Pts',(-0.0157371373481998,-0.575,0.65));
#24956=CARTESIAN_POINT('Ctrl Pts',(-0.0324967135411164,-0.571846918937749,
0.649370620646074));
#24957=CARTESIAN_POINT('Ctrl Pts',(-0.0632828231545123,-0.559077918077178,
0.647096224417991));
#24958=CARTESIAN_POINT('Ctrl Pts',(-0.0773125544088349,-0.549464140887802,
0.645482573914132));
#24959=CARTESIAN_POINT('Ctrl Pts',(-0.099464669894764,-0.527312025401873,
0.642442040715078));
#24960=CARTESIAN_POINT('Ctrl Pts',(-0.109078032552995,-0.513282519396725,
0.640815160902589));
#24961=CARTESIAN_POINT('Ctrl Pts',(-0.121846732641678,-0.482497190457636,
0.63851034608138));
#24962=CARTESIAN_POINT('Ctrl Pts',(-0.125,-0.465737888992352,0.637867541108654));
#24963=CARTESIAN_POINT('Ctrl Pts',(-0.125,-0.45,0.637867541108654));
#24964=CARTESIAN_POINT('Ctrl Pts',(-0.125,-0.45,0.637867541108654));
#24965=CARTESIAN_POINT('Ctrl Pts',(-0.125,-0.434262111007648,0.637867541108654));
#24966=CARTESIAN_POINT('Ctrl Pts',(-0.121846732641678,-0.417502809542363,
0.63851034608138));
#24967=CARTESIAN_POINT('Ctrl Pts',(-0.109078032552995,-0.386717480603274,
0.640815160902589));
#24968=CARTESIAN_POINT('Ctrl Pts',(-0.0994646698947639,-0.372687974598127,
0.642442040715078));
#24969=CARTESIAN_POINT('Ctrl Pts',(-0.0773125544088348,-0.350535859112198,
0.645482573914132));
#24970=CARTESIAN_POINT('Ctrl Pts',(-0.0632828231545122,-0.340922081922822,
0.647096224417991));
#24971=CARTESIAN_POINT('Ctrl Pts',(-0.0324967135411163,-0.328153081062251,
0.649370620646074));
#24972=CARTESIAN_POINT('Ctrl Pts',(-0.0157371373481998,-0.325,0.65));
#24973=CARTESIAN_POINT('Ctrl Pts',(4.5102810375397E-17,-0.325,0.65));
#24974=CARTESIAN_POINT('Origin',(0.,-0.45,0.));
#24975=CARTESIAN_POINT('',(-0.125,-0.45,-0.379967103839267));
#24976=CARTESIAN_POINT('',(-0.125,-0.45,0.));
#24977=CARTESIAN_POINT('',(0.125,-0.45,-0.379967103839267));
#24978=CARTESIAN_POINT('Ctrl Pts',(0.125,-0.45,-0.379967103839267));
#24979=CARTESIAN_POINT('Ctrl Pts',(0.125,-0.465813100629203,-0.379967103839267));
#24980=CARTESIAN_POINT('Ctrl Pts',(0.121817958968287,-0.48260129709332,
-0.381057715344782));
#24981=CARTESIAN_POINT('Ctrl Pts',(0.109029967924066,-0.51336346023721,
-0.384911758361269));
#24982=CARTESIAN_POINT('Ctrl Pts',(0.0994291026068839,-0.527347592689753,
-0.38761064154154));
#24983=CARTESIAN_POINT('Ctrl Pts',(0.0773514949786257,-0.549425200318011,
-0.392612801026882));
#24984=CARTESIAN_POINT('Ctrl Pts',(0.0633657881355918,-0.559029081159106,
-0.395252954914593));
#24985=CARTESIAN_POINT('Ctrl Pts',(0.0325978607437828,-0.571819306519379,
-0.398970551469948));
#24986=CARTESIAN_POINT('Ctrl Pts',(0.0158075115832676,-0.575,-0.4));
#24987=CARTESIAN_POINT('Ctrl Pts',(-0.0158075115832676,-0.575,-0.4));
#24988=CARTESIAN_POINT('Ctrl Pts',(-0.0325978607437828,-0.571819306519379,
-0.398970551469948));
#24989=CARTESIAN_POINT('Ctrl Pts',(-0.0633657881355918,-0.559029081159106,
-0.395252954914593));
#24990=CARTESIAN_POINT('Ctrl Pts',(-0.0773514949786256,-0.549425200318011,
-0.392612801026882));
#24991=CARTESIAN_POINT('Ctrl Pts',(-0.0994291026068839,-0.527347592689753,
-0.38761064154154));
#24992=CARTESIAN_POINT('Ctrl Pts',(-0.109029967924066,-0.51336346023721,
-0.384911758361269));
#24993=CARTESIAN_POINT('Ctrl Pts',(-0.121817958968287,-0.48260129709332,
-0.381057715344782));
#24994=CARTESIAN_POINT('Ctrl Pts',(-0.125,-0.465813100629203,-0.379967103839267));
#24995=CARTESIAN_POINT('Ctrl Pts',(-0.125,-0.45,-0.379967103839267));
#24996=CARTESIAN_POINT('Ctrl Pts',(-0.125,-0.45,-0.379967103839267));
#24997=CARTESIAN_POINT('Ctrl Pts',(-0.125,-0.434186899370797,-0.379967103839267));
#24998=CARTESIAN_POINT('Ctrl Pts',(-0.121817958968287,-0.41739870290668,
-0.381057715344782));
#24999=CARTESIAN_POINT('Ctrl Pts',(-0.109029967924066,-0.38663653976279,
-0.384911758361269));
#25000=CARTESIAN_POINT('Ctrl Pts',(-0.0994291026068839,-0.372652407310247,
-0.38761064154154));
#25001=CARTESIAN_POINT('Ctrl Pts',(-0.0773514949786257,-0.350574799681989,
-0.392612801026882));
#25002=CARTESIAN_POINT('Ctrl Pts',(-0.0633657881355918,-0.340970918840894,
-0.395252954914593));
#25003=CARTESIAN_POINT('Ctrl Pts',(-0.0325978607437829,-0.328180693480621,
-0.398970551469948));
#25004=CARTESIAN_POINT('Ctrl Pts',(-0.0158075115832676,-0.325,-0.4));
#25005=CARTESIAN_POINT('Ctrl Pts',(0.0158075115832675,-0.325,-0.4));
#25006=CARTESIAN_POINT('Ctrl Pts',(0.0325978607437828,-0.328180693480621,
-0.398970551469948));
#25007=CARTESIAN_POINT('Ctrl Pts',(0.0633657881355917,-0.340970918840894,
-0.395252954914593));
#25008=CARTESIAN_POINT('Ctrl Pts',(0.0773514949786256,-0.350574799681989,
-0.392612801026882));
#25009=CARTESIAN_POINT('Ctrl Pts',(0.0994291026068839,-0.372652407310247,
-0.38761064154154));
#25010=CARTESIAN_POINT('Ctrl Pts',(0.109029967924066,-0.38663653976279,
-0.384911758361269));
#25011=CARTESIAN_POINT('Ctrl Pts',(0.121817958968287,-0.41739870290668,
-0.381057715344782));
#25012=CARTESIAN_POINT('Ctrl Pts',(0.125,-0.434186899370797,-0.379967103839267));
#25013=CARTESIAN_POINT('Ctrl Pts',(0.125,-0.45,-0.379967103839267));
#25014=CARTESIAN_POINT('Origin',(0.,-0.45,0.));
#25015=CARTESIAN_POINT('',(0.125,-0.45,0.379967103839267));
#25016=CARTESIAN_POINT('',(-0.125,-0.45,0.379967103839267));
#25017=CARTESIAN_POINT('Ctrl Pts',(0.125,-0.45,0.379967103839267));
#25018=CARTESIAN_POINT('Ctrl Pts',(0.125,-0.434186899370797,0.379967103839267));
#25019=CARTESIAN_POINT('Ctrl Pts',(0.121817958968287,-0.41739870290668,
0.381057715344782));
#25020=CARTESIAN_POINT('Ctrl Pts',(0.109029967924066,-0.38663653976279,
0.384911758361269));
#25021=CARTESIAN_POINT('Ctrl Pts',(0.0994291026068839,-0.372652407310247,
0.38761064154154));
#25022=CARTESIAN_POINT('Ctrl Pts',(0.0773514949786256,-0.350574799681989,
0.392612801026882));
#25023=CARTESIAN_POINT('Ctrl Pts',(0.0633657881355918,-0.340970918840894,
0.395252954914593));
#25024=CARTESIAN_POINT('Ctrl Pts',(0.0325978607437828,-0.328180693480621,
0.398970551469948));
#25025=CARTESIAN_POINT('Ctrl Pts',(0.0158075115832676,-0.325,0.4));
#25026=CARTESIAN_POINT('Ctrl Pts',(-0.0158075115832676,-0.325,0.4));
#25027=CARTESIAN_POINT('Ctrl Pts',(-0.0325978607437828,-0.328180693480621,
0.398970551469948));
#25028=CARTESIAN_POINT('Ctrl Pts',(-0.0633657881355918,-0.340970918840894,
0.395252954914593));
#25029=CARTESIAN_POINT('Ctrl Pts',(-0.0773514949786257,-0.350574799681989,
0.392612801026882));
#25030=CARTESIAN_POINT('Ctrl Pts',(-0.0994291026068839,-0.372652407310247,
0.38761064154154));
#25031=CARTESIAN_POINT('Ctrl Pts',(-0.109029967924066,-0.38663653976279,
0.384911758361269));
#25032=CARTESIAN_POINT('Ctrl Pts',(-0.121817958968287,-0.41739870290668,
0.381057715344782));
#25033=CARTESIAN_POINT('Ctrl Pts',(-0.125,-0.434186899370797,0.379967103839267));
#25034=CARTESIAN_POINT('Ctrl Pts',(-0.125,-0.45,0.379967103839267));
#25035=CARTESIAN_POINT('Ctrl Pts',(-0.125,-0.45,0.379967103839267));
#25036=CARTESIAN_POINT('Ctrl Pts',(-0.125,-0.465813100629203,0.379967103839267));
#25037=CARTESIAN_POINT('Ctrl Pts',(-0.121817958968287,-0.48260129709332,
0.381057715344782));
#25038=CARTESIAN_POINT('Ctrl Pts',(-0.109029967924066,-0.51336346023721,
0.384911758361269));
#25039=CARTESIAN_POINT('Ctrl Pts',(-0.0994291026068839,-0.527347592689753,
0.38761064154154));
#25040=CARTESIAN_POINT('Ctrl Pts',(-0.0773514949786256,-0.549425200318011,
0.392612801026882));
#25041=CARTESIAN_POINT('Ctrl Pts',(-0.0633657881355917,-0.559029081159106,
0.395252954914593));
#25042=CARTESIAN_POINT('Ctrl Pts',(-0.0325978607437828,-0.571819306519379,
0.398970551469948));
#25043=CARTESIAN_POINT('Ctrl Pts',(-0.0158075115832675,-0.575,0.4));
#25044=CARTESIAN_POINT('Ctrl Pts',(0.0158075115832676,-0.575,0.4));
#25045=CARTESIAN_POINT('Ctrl Pts',(0.0325978607437828,-0.571819306519379,
0.398970551469948));
#25046=CARTESIAN_POINT('Ctrl Pts',(0.0633657881355917,-0.559029081159106,
0.395252954914593));
#25047=CARTESIAN_POINT('Ctrl Pts',(0.0773514949786257,-0.549425200318011,
0.392612801026882));
#25048=CARTESIAN_POINT('Ctrl Pts',(0.0994291026068839,-0.527347592689753,
0.38761064154154));
#25049=CARTESIAN_POINT('Ctrl Pts',(0.109029967924066,-0.51336346023721,
0.384911758361269));
#25050=CARTESIAN_POINT('Ctrl Pts',(0.121817958968287,-0.48260129709332,
0.381057715344782));
#25051=CARTESIAN_POINT('Ctrl Pts',(0.125,-0.465813100629203,0.379967103839267));
#25052=CARTESIAN_POINT('Ctrl Pts',(0.125,-0.45,0.379967103839267));
#25053=CARTESIAN_POINT('',(-0.125,-0.45,0.));
#25054=CARTESIAN_POINT('Origin',(0.,0.,0.));
#25055=CARTESIAN_POINT('',(-0.4,-0.8,4.89858719658941E-17));
#25056=CARTESIAN_POINT('Origin',(0.,-0.8,0.));
#25057=CARTESIAN_POINT('',(-0.4,0.,4.89858719658941E-17));
#25058=CARTESIAN_POINT('',(-0.4,0.85,-4.89858719658941E-17));
#25059=CARTESIAN_POINT('',(-0.4,0.,4.89858719658941E-17));
#25060=CARTESIAN_POINT('Origin',(0.,0.85,0.));
#25061=CARTESIAN_POINT('Origin',(0.,-0.8,0.));
#25062=CARTESIAN_POINT('Origin',(0.,0.,0.));
#25063=CARTESIAN_POINT('',(-0.8,0.,9.79717439317883E-17));
#25064=CARTESIAN_POINT('Origin',(0.,0.,0.));
#25065=CARTESIAN_POINT('',(0.595438916863769,0.,0.137993139022126));
#25066=CARTESIAN_POINT('',(0.562830534889751,0.,0.238351419397483));
#25067=CARTESIAN_POINT('Origin',(0.562758945330873,0.,0.182851465569258));
#25068=CARTESIAN_POINT('',(0.523653836874034,0.,0.315240018494132));
#25069=CARTESIAN_POINT('Origin',(0.,0.,0.));
#25070=CARTESIAN_POINT('',(0.461629008549572,0.,0.40060987082025));
#25071=CARTESIAN_POINT('Origin',(0.478711351753049,0.,0.347804155687524));
#25072=CARTESIAN_POINT('',(0.40060987082025,0.,0.461629008549572));
#25073=CARTESIAN_POINT('Origin',(0.,0.,0.));
#25074=CARTESIAN_POINT('',(0.315240018494132,0.,0.523653836874034));
#25075=CARTESIAN_POINT('Origin',(0.347804155687523,0.,0.478711351753049));
#25076=CARTESIAN_POINT('',(0.238351419397483,0.,0.562830534889751));
#25077=CARTESIAN_POINT('Origin',(0.,0.,0.));
#25078=CARTESIAN_POINT('',(0.137993139022126,0.,0.595438916863769));
#25079=CARTESIAN_POINT('Origin',(0.182851465569258,0.,0.562758945330873));
#25080=CARTESIAN_POINT('',(0.0527614703521001,0.,0.608938287003997));
#25081=CARTESIAN_POINT('Origin',(0.,0.,0.));
#25082=CARTESIAN_POINT('',(-0.0527614703521003,0.,0.608938287003997));
#25083=CARTESIAN_POINT('Origin',(-1.08697158783324E-16,0.,0.591719772367581));
#25084=CARTESIAN_POINT('',(-0.137993139022126,0.,0.595438916863769));
#25085=CARTESIAN_POINT('Origin',(0.,0.,0.));
#25086=CARTESIAN_POINT('',(-0.238351419397483,0.,0.562830534889751));
#25087=CARTESIAN_POINT('Origin',(-0.182851465569258,0.,0.562758945330873));
#25088=CARTESIAN_POINT('',(-0.315240018494132,0.,0.523653836874034));
#25089=CARTESIAN_POINT('Origin',(0.,0.,0.));
#25090=CARTESIAN_POINT('',(-0.40060987082025,0.,0.461629008549572));
#25091=CARTESIAN_POINT('Origin',(-0.347804155687524,0.,0.478711351753049));
#25092=CARTESIAN_POINT('',(-0.461629008549572,0.,0.40060987082025));
#25093=CARTESIAN_POINT('Origin',(0.,0.,0.));
#25094=CARTESIAN_POINT('',(-0.523653836874034,0.,0.315240018494132));
#25095=CARTESIAN_POINT('Origin',(-0.478711351753049,0.,0.347804155687524));
#25096=CARTESIAN_POINT('',(-0.562830534889751,0.,0.238351419397483));
#25097=CARTESIAN_POINT('Origin',(0.,0.,0.));
#25098=CARTESIAN_POINT('',(-0.595438916863769,0.,0.137993139022126));
#25099=CARTESIAN_POINT('Origin',(-0.562758945330873,0.,0.182851465569258));
#25100=CARTESIAN_POINT('',(-0.608938287003997,0.,0.0527614703521002));
#25101=CARTESIAN_POINT('Origin',(0.,0.,0.));
#25102=CARTESIAN_POINT('',(-0.608938287003997,0.,-0.0527614703521003));
#25103=CARTESIAN_POINT('Origin',(-0.591719772367581,0.,-7.24647725222159E-17));
#25104=CARTESIAN_POINT('',(-0.595438916863769,0.,-0.137993139022126));
#25105=CARTESIAN_POINT('Origin',(0.,0.,0.));
#25106=CARTESIAN_POINT('',(-0.562830534889751,0.,-0.238351419397483));
#25107=CARTESIAN_POINT('Origin',(-0.562758945330873,0.,-0.182851465569258));
#25108=CARTESIAN_POINT('',(-0.523653836874034,0.,-0.315240018494132));
#25109=CARTESIAN_POINT('Origin',(0.,0.,0.));
#25110=CARTESIAN_POINT('',(-0.461629008549572,0.,-0.40060987082025));
#25111=CARTESIAN_POINT('Origin',(-0.478711351753049,0.,-0.347804155687524));
#25112=CARTESIAN_POINT('',(-0.40060987082025,0.,-0.461629008549572));
#25113=CARTESIAN_POINT('Origin',(0.,0.,0.));
#25114=CARTESIAN_POINT('',(-0.315240018494132,0.,-0.523653836874034));
#25115=CARTESIAN_POINT('Origin',(-0.347804155687524,0.,-0.478711351753049));
#25116=CARTESIAN_POINT('',(-0.238351419397483,0.,-0.562830534889751));
#25117=CARTESIAN_POINT('Origin',(0.,0.,0.));
#25118=CARTESIAN_POINT('',(-0.137993139022126,0.,-0.595438916863769));
#25119=CARTESIAN_POINT('Origin',(-0.182851465569258,0.,-0.562758945330873));
#25120=CARTESIAN_POINT('',(-0.0527614703521002,0.,-0.608938287003997));
#25121=CARTESIAN_POINT('Origin',(0.,0.,0.));
#25122=CARTESIAN_POINT('',(0.0527614703521003,0.,-0.608938287003997));
#25123=CARTESIAN_POINT('Origin',(3.6232386261108E-17,0.,-0.591719772367581));
#25124=CARTESIAN_POINT('',(0.137993139022126,0.,-0.595438916863769));
#25125=CARTESIAN_POINT('Origin',(0.,0.,0.));
#25126=CARTESIAN_POINT('',(0.238351419397483,0.,-0.562830534889751));
#25127=CARTESIAN_POINT('Origin',(0.182851465569258,0.,-0.562758945330873));
#25128=CARTESIAN_POINT('',(0.315240018494132,0.,-0.523653836874034));
#25129=CARTESIAN_POINT('Origin',(0.,0.,0.));
#25130=CARTESIAN_POINT('',(0.40060987082025,0.,-0.461629008549572));
#25131=CARTESIAN_POINT('Origin',(0.347804155687524,0.,-0.478711351753049));
#25132=CARTESIAN_POINT('',(0.461629008549572,0.,-0.40060987082025));
#25133=CARTESIAN_POINT('Origin',(0.,0.,0.));
#25134=CARTESIAN_POINT('',(0.523653836874034,0.,-0.315240018494132));
#25135=CARTESIAN_POINT('Origin',(0.478711351753049,0.,-0.347804155687524));
#25136=CARTESIAN_POINT('',(0.562830534889751,0.,-0.238351419397483));
#25137=CARTESIAN_POINT('Origin',(0.,0.,0.));
#25138=CARTESIAN_POINT('',(0.595438916863769,0.,-0.137993139022126));
#25139=CARTESIAN_POINT('Origin',(0.562758945330873,0.,-0.182851465569258));
#25140=CARTESIAN_POINT('',(0.608938287003997,0.,-0.0527614703521001));
#25141=CARTESIAN_POINT('Origin',(0.,0.,0.));
#25142=CARTESIAN_POINT('',(0.608938287003997,0.,0.0527614703521001));
#25143=CARTESIAN_POINT('Origin',(0.591719772367581,0.,0.));
#25144=CARTESIAN_POINT('Origin',(0.,0.,0.));
#25145=CARTESIAN_POINT('Origin',(0.,0.,0.));
#25146=CARTESIAN_POINT('',(-0.8,-0.1,9.79717439317883E-17));
#25147=CARTESIAN_POINT('Origin',(0.,-0.1,0.));
#25148=CARTESIAN_POINT('',(-0.8,0.,-9.79717439317883E-17));
#25149=CARTESIAN_POINT('Origin',(0.,-0.1,0.));
#25150=CARTESIAN_POINT('Origin',(0.,0.75,0.));
#25151=CARTESIAN_POINT('',(-0.8,0.75,9.79717439317883E-17));
#25152=CARTESIAN_POINT('Origin',(0.,0.75,0.));
#25153=CARTESIAN_POINT('',(0.562830534889751,0.75,0.238351419397483));
#25154=CARTESIAN_POINT('',(0.595438916863769,0.75,0.137993139022126));
#25155=CARTESIAN_POINT('Origin',(0.562758945330873,0.75,0.182851465569258));
#25156=CARTESIAN_POINT('',(0.608938287003997,0.75,0.0527614703521002));
#25157=CARTESIAN_POINT('Origin',(0.,0.75,0.));
#25158=CARTESIAN_POINT('',(0.608938287003997,0.75,-0.0527614703521002));
#25159=CARTESIAN_POINT('Origin',(0.591719772367581,0.75,0.));
#25160=CARTESIAN_POINT('',(0.595438916863769,0.75,-0.137993139022126));
#25161=CARTESIAN_POINT('Origin',(0.,0.75,0.));
#25162=CARTESIAN_POINT('',(0.562830534889751,0.75,-0.238351419397483));
#25163=CARTESIAN_POINT('Origin',(0.562758945330873,0.75,-0.182851465569258));
#25164=CARTESIAN_POINT('',(0.523653836874034,0.75,-0.315240018494132));
#25165=CARTESIAN_POINT('Origin',(0.,0.75,0.));
#25166=CARTESIAN_POINT('',(0.461629008549572,0.75,-0.40060987082025));
#25167=CARTESIAN_POINT('Origin',(0.478711351753049,0.75,-0.347804155687524));
#25168=CARTESIAN_POINT('',(0.40060987082025,0.75,-0.461629008549572));
#25169=CARTESIAN_POINT('Origin',(0.,0.75,0.));
#25170=CARTESIAN_POINT('',(0.315240018494132,0.75,-0.523653836874034));
#25171=CARTESIAN_POINT('Origin',(0.347804155687524,0.75,-0.478711351753049));
#25172=CARTESIAN_POINT('',(0.238351419397483,0.75,-0.562830534889751));
#25173=CARTESIAN_POINT('Origin',(0.,0.75,0.));
#25174=CARTESIAN_POINT('',(0.137993139022126,0.75,-0.595438916863769));
#25175=CARTESIAN_POINT('Origin',(0.182851465569258,0.75,-0.562758945330873));
#25176=CARTESIAN_POINT('',(0.0527614703521003,0.75,-0.608938287003997));
#25177=CARTESIAN_POINT('Origin',(0.,0.75,0.));
#25178=CARTESIAN_POINT('',(-0.0527614703521002,0.75,-0.608938287003997));
#25179=CARTESIAN_POINT('Origin',(3.6232386261108E-17,0.75,-0.591719772367581));
#25180=CARTESIAN_POINT('',(-0.137993139022126,0.75,-0.595438916863769));
#25181=CARTESIAN_POINT('Origin',(0.,0.75,0.));
#25182=CARTESIAN_POINT('',(-0.238351419397483,0.75,-0.562830534889751));
#25183=CARTESIAN_POINT('Origin',(-0.182851465569258,0.75,-0.562758945330873));
#25184=CARTESIAN_POINT('',(-0.315240018494132,0.75,-0.523653836874034));
#25185=CARTESIAN_POINT('Origin',(0.,0.75,0.));
#25186=CARTESIAN_POINT('',(-0.40060987082025,0.75,-0.461629008549572));
#25187=CARTESIAN_POINT('Origin',(-0.347804155687524,0.75,-0.478711351753049));
#25188=CARTESIAN_POINT('',(-0.461629008549572,0.75,-0.40060987082025));
#25189=CARTESIAN_POINT('Origin',(0.,0.75,0.));
#25190=CARTESIAN_POINT('',(-0.523653836874034,0.75,-0.315240018494132));
#25191=CARTESIAN_POINT('Origin',(-0.478711351753049,0.75,-0.347804155687524));
#25192=CARTESIAN_POINT('',(-0.562830534889751,0.75,-0.238351419397483));
#25193=CARTESIAN_POINT('Origin',(0.,0.75,0.));
#25194=CARTESIAN_POINT('',(-0.595438916863769,0.75,-0.137993139022126));
#25195=CARTESIAN_POINT('Origin',(-0.562758945330873,0.75,-0.182851465569258));
#25196=CARTESIAN_POINT('',(-0.608938287003997,0.75,-0.0527614703521003));
#25197=CARTESIAN_POINT('Origin',(0.,0.75,0.));
#25198=CARTESIAN_POINT('',(-0.608938287003997,0.75,0.0527614703521002));
#25199=CARTESIAN_POINT('Origin',(-0.591719772367581,0.75,-7.24647725222159E-17));
#25200=CARTESIAN_POINT('',(-0.595438916863769,0.75,0.137993139022126));
#25201=CARTESIAN_POINT('Origin',(0.,0.75,0.));
#25202=CARTESIAN_POINT('',(-0.562830534889751,0.75,0.238351419397483));
#25203=CARTESIAN_POINT('Origin',(-0.562758945330873,0.75,0.182851465569258));
#25204=CARTESIAN_POINT('',(-0.523653836874034,0.75,0.315240018494132));
#25205=CARTESIAN_POINT('Origin',(0.,0.75,0.));
#25206=CARTESIAN_POINT('',(-0.461629008549572,0.75,0.40060987082025));
#25207=CARTESIAN_POINT('Origin',(-0.478711351753049,0.75,0.347804155687524));
#25208=CARTESIAN_POINT('',(-0.40060987082025,0.75,0.461629008549572));
#25209=CARTESIAN_POINT('Origin',(0.,0.75,0.));
#25210=CARTESIAN_POINT('',(-0.315240018494132,0.75,0.523653836874034));
#25211=CARTESIAN_POINT('Origin',(-0.347804155687524,0.75,0.478711351753049));
#25212=CARTESIAN_POINT('',(-0.238351419397483,0.75,0.562830534889751));
#25213=CARTESIAN_POINT('Origin',(0.,0.75,0.));
#25214=CARTESIAN_POINT('',(-0.137993139022126,0.75,0.595438916863769));
#25215=CARTESIAN_POINT('Origin',(-0.182851465569258,0.75,0.562758945330873));
#25216=CARTESIAN_POINT('',(-0.0527614703521003,0.75,0.608938287003997));
#25217=CARTESIAN_POINT('Origin',(0.,0.75,0.));
#25218=CARTESIAN_POINT('',(0.0527614703521001,0.75,0.608938287003997));
#25219=CARTESIAN_POINT('Origin',(-1.08697158783324E-16,0.75,0.591719772367581));
#25220=CARTESIAN_POINT('',(0.137993139022126,0.75,0.595438916863769));
#25221=CARTESIAN_POINT('Origin',(0.,0.75,0.));
#25222=CARTESIAN_POINT('',(0.238351419397483,0.75,0.562830534889751));
#25223=CARTESIAN_POINT('Origin',(0.182851465569258,0.75,0.562758945330873));
#25224=CARTESIAN_POINT('',(0.315240018494132,0.75,0.523653836874034));
#25225=CARTESIAN_POINT('Origin',(0.,0.75,0.));
#25226=CARTESIAN_POINT('',(0.40060987082025,0.75,0.461629008549572));
#25227=CARTESIAN_POINT('Origin',(0.347804155687523,0.75,0.478711351753049));
#25228=CARTESIAN_POINT('',(0.461629008549572,0.75,0.40060987082025));
#25229=CARTESIAN_POINT('Origin',(0.,0.75,0.));
#25230=CARTESIAN_POINT('',(0.523653836874034,0.75,0.315240018494132));
#25231=CARTESIAN_POINT('Origin',(0.478711351753049,0.75,0.347804155687524));
#25232=CARTESIAN_POINT('Origin',(0.,0.75,0.));
#25233=CARTESIAN_POINT('Origin',(0.,0.75,0.));
#25234=CARTESIAN_POINT('',(-0.8,0.85,9.79717439317883E-17));
#25235=CARTESIAN_POINT('Origin',(0.,0.85,0.));
#25236=CARTESIAN_POINT('',(-0.8,0.75,9.79717439317883E-17));
#25237=CARTESIAN_POINT('Origin',(0.,0.85,0.));
#25238=CARTESIAN_POINT('Origin',(0.562758945330873,0.,0.182851465569258));
#25239=CARTESIAN_POINT('',(0.595438916863769,0.,0.137993139022126));
#25240=CARTESIAN_POINT('',(0.562830534889751,0.,0.238351419397483));
#25241=CARTESIAN_POINT('Origin',(0.,0.,0.));
#25242=CARTESIAN_POINT('',(0.523653836874034,0.,0.315240018494132));
#25243=CARTESIAN_POINT('Origin',(0.478711351753049,0.,0.347804155687524));
#25244=CARTESIAN_POINT('',(0.461629008549572,0.,0.40060987082025));
#25245=CARTESIAN_POINT('Origin',(0.,0.,0.));
#25246=CARTESIAN_POINT('',(0.40060987082025,0.,0.461629008549572));
#25247=CARTESIAN_POINT('Origin',(0.347804155687523,0.,0.478711351753049));
#25248=CARTESIAN_POINT('',(0.315240018494132,0.,0.523653836874034));
#25249=CARTESIAN_POINT('Origin',(0.,0.,0.));
#25250=CARTESIAN_POINT('',(0.238351419397483,0.,0.562830534889751));
#25251=CARTESIAN_POINT('Origin',(0.182851465569258,0.,0.562758945330873));
#25252=CARTESIAN_POINT('',(0.137993139022126,0.,0.595438916863769));
#25253=CARTESIAN_POINT('Origin',(0.,0.,0.));
#25254=CARTESIAN_POINT('',(0.0527614703521,0.,0.608938287003997));
#25255=CARTESIAN_POINT('Origin',(-1.08697158783324E-16,0.,0.591719772367581));
#25256=CARTESIAN_POINT('',(-0.0527614703521002,0.,0.608938287003997));
#25257=CARTESIAN_POINT('Origin',(0.,0.,0.));
#25258=CARTESIAN_POINT('',(-0.137993139022126,0.,0.595438916863769));
#25259=CARTESIAN_POINT('Origin',(-0.182851465569258,0.,0.562758945330873));
#25260=CARTESIAN_POINT('',(-0.238351419397483,0.,0.562830534889751));
#25261=CARTESIAN_POINT('Origin',(0.,0.,0.));
#25262=CARTESIAN_POINT('',(-0.315240018494132,0.,0.523653836874034));
#25263=CARTESIAN_POINT('Origin',(-0.347804155687524,0.,0.478711351753049));
#25264=CARTESIAN_POINT('',(-0.40060987082025,0.,0.461629008549572));
#25265=CARTESIAN_POINT('Origin',(0.,0.,0.));
#25266=CARTESIAN_POINT('',(-0.461629008549572,0.,0.40060987082025));
#25267=CARTESIAN_POINT('Origin',(-0.478711351753049,0.,0.347804155687524));
#25268=CARTESIAN_POINT('',(-0.523653836874034,0.,0.315240018494132));
#25269=CARTESIAN_POINT('Origin',(0.,0.,0.));
#25270=CARTESIAN_POINT('',(-0.562830534889751,0.,0.238351419397483));
#25271=CARTESIAN_POINT('Origin',(-0.562758945330873,0.,0.182851465569258));
#25272=CARTESIAN_POINT('',(-0.595438916863769,0.,0.137993139022126));
#25273=CARTESIAN_POINT('Origin',(0.,0.,0.));
#25274=CARTESIAN_POINT('',(-0.608938287003997,0.,0.0527614703521));
#25275=CARTESIAN_POINT('Origin',(-0.591719772367581,0.,-7.24647725222159E-17));
#25276=CARTESIAN_POINT('',(-0.608938287003997,0.,-0.0527614703521002));
#25277=CARTESIAN_POINT('Origin',(0.,0.,0.));
#25278=CARTESIAN_POINT('',(-0.595438916863769,0.,-0.137993139022126));
#25279=CARTESIAN_POINT('Origin',(-0.562758945330873,0.,-0.182851465569258));
#25280=CARTESIAN_POINT('',(-0.562830534889751,0.,-0.238351419397483));
#25281=CARTESIAN_POINT('Origin',(0.,0.,0.));
#25282=CARTESIAN_POINT('',(-0.523653836874034,0.,-0.315240018494132));
#25283=CARTESIAN_POINT('Origin',(-0.478711351753049,0.,-0.347804155687524));
#25284=CARTESIAN_POINT('',(-0.461629008549572,0.,-0.40060987082025));
#25285=CARTESIAN_POINT('Origin',(0.,0.,0.));
#25286=CARTESIAN_POINT('',(-0.40060987082025,0.,-0.461629008549572));
#25287=CARTESIAN_POINT('Origin',(-0.347804155687524,0.,-0.478711351753049));
#25288=CARTESIAN_POINT('',(-0.315240018494132,0.,-0.523653836874034));
#25289=CARTESIAN_POINT('Origin',(0.,0.,0.));
#25290=CARTESIAN_POINT('',(-0.238351419397483,0.,-0.562830534889751));
#25291=CARTESIAN_POINT('Origin',(-0.182851465569258,0.,-0.562758945330873));
#25292=CARTESIAN_POINT('',(-0.137993139022126,0.,-0.595438916863769));
#25293=CARTESIAN_POINT('Origin',(0.,0.,0.));
#25294=CARTESIAN_POINT('',(-0.0527614703521,0.,-0.608938287003997));
#25295=CARTESIAN_POINT('Origin',(3.6232386261108E-17,0.,-0.591719772367581));
#25296=CARTESIAN_POINT('',(0.0527614703521001,0.,-0.608938287003997));
#25297=CARTESIAN_POINT('Origin',(0.,0.,0.));
#25298=CARTESIAN_POINT('',(0.137993139022126,0.,-0.595438916863769));
#25299=CARTESIAN_POINT('Origin',(0.182851465569258,0.,-0.562758945330873));
#25300=CARTESIAN_POINT('',(0.238351419397483,0.,-0.562830534889751));
#25301=CARTESIAN_POINT('Origin',(0.,0.,0.));
#25302=CARTESIAN_POINT('',(0.315240018494132,0.,-0.523653836874034));
#25303=CARTESIAN_POINT('Origin',(0.347804155687524,0.,-0.478711351753049));
#25304=CARTESIAN_POINT('',(0.40060987082025,0.,-0.461629008549572));
#25305=CARTESIAN_POINT('Origin',(0.,0.,0.));
#25306=CARTESIAN_POINT('',(0.461629008549572,0.,-0.40060987082025));
#25307=CARTESIAN_POINT('Origin',(0.478711351753049,0.,-0.347804155687524));
#25308=CARTESIAN_POINT('',(0.523653836874034,0.,-0.315240018494132));
#25309=CARTESIAN_POINT('Origin',(0.,0.,0.));
#25310=CARTESIAN_POINT('',(0.562830534889751,0.,-0.238351419397483));
#25311=CARTESIAN_POINT('Origin',(0.562758945330873,0.,-0.182851465569258));
#25312=CARTESIAN_POINT('',(0.595438916863769,0.,-0.137993139022126));
#25313=CARTESIAN_POINT('Origin',(0.,0.,0.));
#25314=CARTESIAN_POINT('',(0.608938287003997,0.,0.0527614703521001));
#25315=CARTESIAN_POINT('Origin',(0.591719772367581,0.,0.));
#25316=CARTESIAN_POINT('',(0.608938287003997,0.,-0.0527614703521001));
#25317=CARTESIAN_POINT('Origin',(0.,0.,0.));
#26974=UNCERTAINTY_MEASURE_WITH_UNIT(LENGTH_MEASURE(0.001),#27070,
'DISTANCE_ACCURACY_VALUE',
'Maximum model space distance between geometric entities at asserted c
onnectivities');
#26992=UNCERTAINTY_MEASURE_WITH_UNIT(LENGTH_MEASURE(0.001),#27070,
'DISTANCE_ACCURACY_VALUE',
'Maximum model space distance between geometric entities at asserted c
onnectivities');
#27051=(
GEOMETRIC_REPRESENTATION_CONTEXT(3)
GLOBAL_UNCERTAINTY_ASSIGNED_CONTEXT((#26974))
GLOBAL_UNIT_ASSIGNED_CONTEXT((#27070,#27072,#27073))
REPRESENTATION_CONTEXT('','3D')
);
#27069=(
GEOMETRIC_REPRESENTATION_CONTEXT(3)
GLOBAL_UNCERTAINTY_ASSIGNED_CONTEXT((#26992))
GLOBAL_UNIT_ASSIGNED_CONTEXT((#27070,#27072,#27073))
REPRESENTATION_CONTEXT('','3D')
);
#27070=(
LENGTH_UNIT()
NAMED_UNIT(*)
SI_UNIT(.CENTI.,.METRE.)
);
#27072=(
NAMED_UNIT(*)
PLANE_ANGLE_UNIT()
SI_UNIT($,.RADIAN.)
);
#27073=(
NAMED_UNIT(*)
SI_UNIT($,.STERADIAN.)
SOLID_ANGLE_UNIT()
);
#27132=SHAPE_DEFINITION_REPRESENTATION(#27220,#27409);
#27220=PRODUCT_DEFINITION_SHAPE('',$,#27486);
#27409=SHAPE_REPRESENTATION('',(#15729),#27051);
#27427=PRODUCT_DEFINITION_CONTEXT('part definition',#27657,'design');
#27486=PRODUCT_DEFINITION(
'Timing Pulley - 2 mm Pitch, 20 Teeth, 8 mm Bore',
'Timing Pulley - 2 mm Pitch, 20 Teeth, 8 mm Bore',#27562,#27427);
#27562=PRODUCT_DEFINITION_FORMATION('',$,#27717);
#27657=APPLICATION_CONTEXT(
'Core Data for Automotive Mechanical Design Process');
#27658=PRODUCT_CONTEXT('part definition',#27657,'mechanical');
#27717=PRODUCT('Timing Pulley - 2 mm Pitch, 20 Teeth, 8 mm Bore',
'Timing Pulley - 2 mm Pitch, 20 Teeth, 8 mm Bore',
'Timing Pulley - 2 mm Pitch, 20 Teeth, 8 mm Bore',(#27658));
#27805=COLOUR_RGB('Off White',0.89,0.88,0.83);
#27806=FILL_AREA_STYLE_COLOUR('',#27805);
#27807=FILL_AREA_STYLE('',(#27806));
#27808=SURFACE_STYLE_FILL_AREA(#27807);
#27809=SURFACE_SIDE_STYLE('',(#27808));
#27810=SURFACE_STYLE_USAGE(.BOTH.,#27809);
#27811=PRESENTATION_STYLE_ASSIGNMENT((#27810));
ENDSEC;
END-ISO-10303-21;
